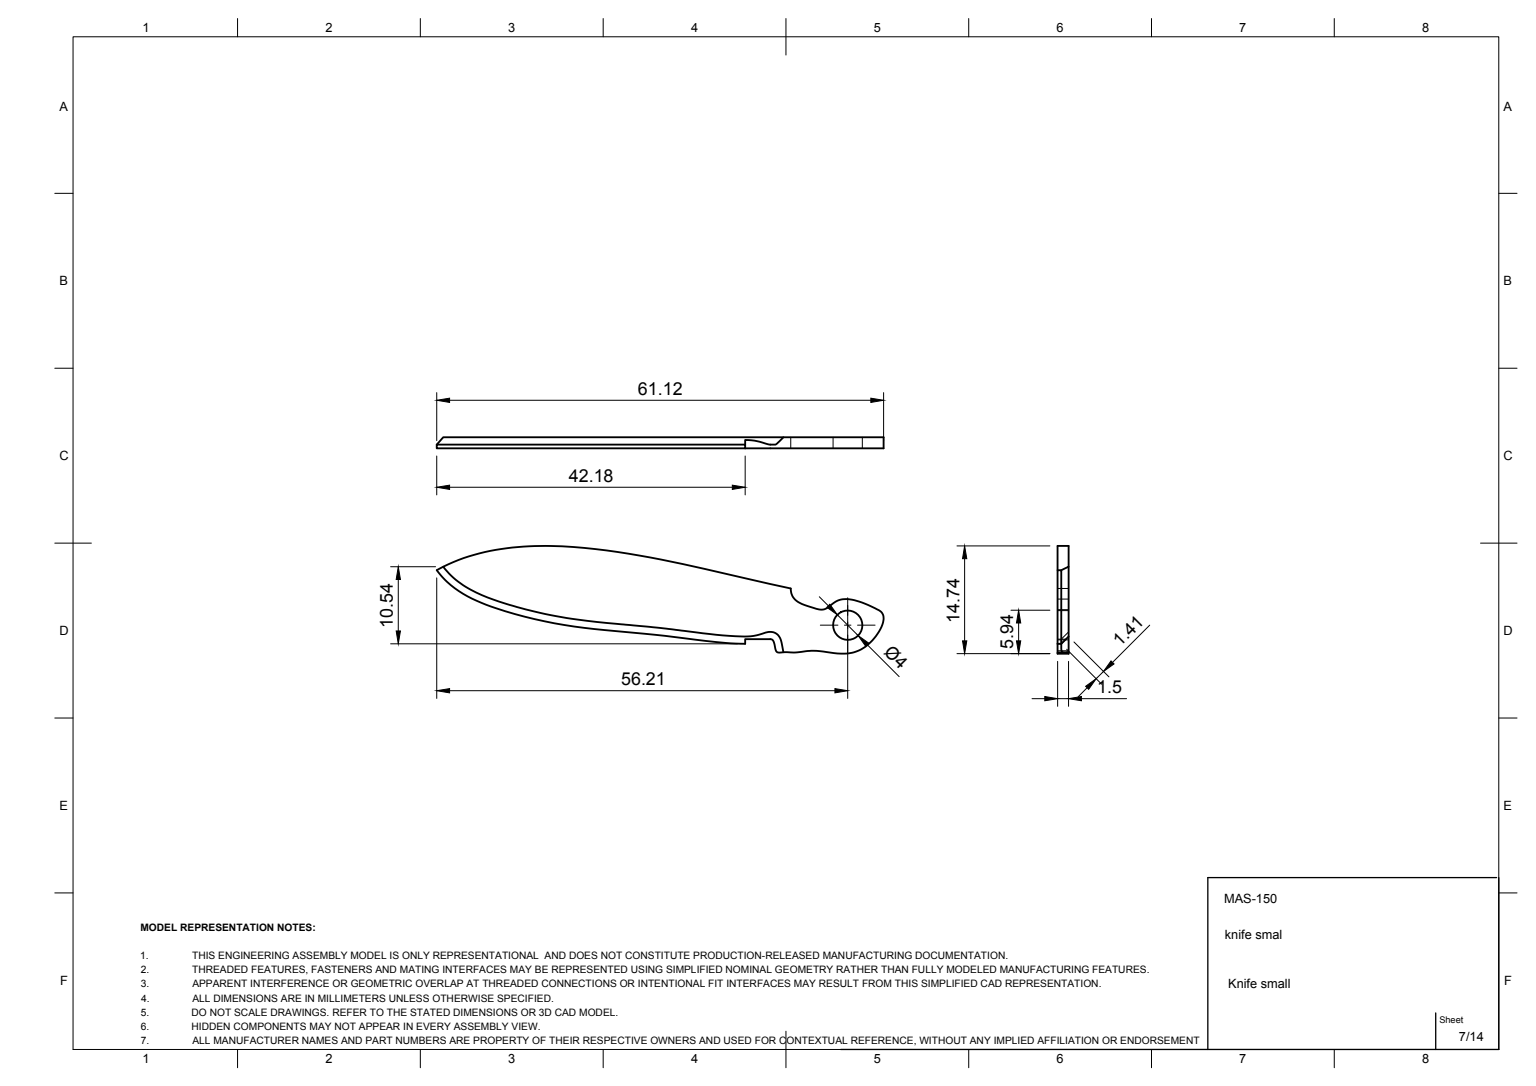
ISO-10303-21;
HEADER;
/* Generated by software containing ST-Developer
 * from STEP Tools, Inc. (www.steptools.com) 
 */

FILE_DESCRIPTION(
/* description */ ('STEP AP203'),
/* implementation_level */ '2;1');

FILE_NAME(
/* name */ 'Knife small.step',
/* time_stamp */ '2026-11-08T21:40:52-08:00',
/* author */ (''),
/* organization */ (''),
/* preprocessor_version */ 'ST-DEVELOPER v20.2',
/* originating_system */ 'Autodesk Translation Framework v15.17.0.0',
/* authorisation */ '');

FILE_SCHEMA (('AUTOMOTIVE_DESIGN { 1 0 10303 214 3 1 1 }'));
ENDSEC;

DATA;
#10=MECHANICAL_DESIGN_GEOMETRIC_PRESENTATION_REPRESENTATION('',(#185),#12137);
#91=B_SPLINE_CURVE_WITH_KNOTS('',3,(#3645,#3646,#3647,#3648,#3649,#3650,
#3651,#3652),.UNSPECIFIED.,.F.,.F.,(4,1,1,1,1,4),(0.,0.0142399187551309,
0.253552302413509,0.548288200579205,0.757181970713106,0.999999999751732),
 .UNSPECIFIED.);
#92=B_SPLINE_CURVE_WITH_KNOTS('',3,(#3655,#3656,#3657,#3658,#3659,#3660,
#3661,#3662),.UNSPECIFIED.,.F.,.F.,(4,1,1,1,1,4),(0.,0.156258367612318,
0.290685780689375,0.48035435867502,0.63435677163295,0.643520450566124),
 .UNSPECIFIED.);
#93=B_SPLINE_CURVE_WITH_KNOTS('',3,(#3689,#3690,#3691,#3692,#3693,#3694,
#3695,#3696),.UNSPECIFIED.,.F.,.F.,(4,1,1,1,1,4),(0.736469307506587,0.759577826910316,
0.780092040409136,0.810242072545427,0.901462701662728,0.958125874426747),
 .UNSPECIFIED.);
#94=B_SPLINE_CURVE_WITH_KNOTS('',3,(#3698,#3699,#3700,#3701,#3702,#3703,
#3704,#3705,#3706,#3707,#3708,#3709,#3710,#3711,#3712,#3713,#3714,#3715,
#3716,#3717,#3718,#3719,#3720,#3721,#3722,#3723,#3724,#3725,#3726,#3727,
#3728,#3729,#3730,#3731,#3732,#3733,#3734,#3735,#3736,#3737,#3738,#3739,
#3740,#3741,#3742,#3743,#3744,#3745,#3746,#3747,#3748,#3749,#3750,#3751,
#3752,#3753,#3754,#3755,#3756,#3757,#3758,#3759,#3760,#3761,#3762,#3763,
#3764,#3765,#3766,#3767,#3768,#3769,#3770,#3771,#3772,#3773,#3774,#3775,
#3776,#3777,#3778,#3779,#3780,#3781,#3782,#3783,#3784,#3785,#3786,#3787,
#3788,#3789,#3790,#3791,#3792,#3793,#3794,#3795,#3796,#3797,#3798,#3799,
#3800,#3801,#3802,#3803,#3804,#3805,#3806,#3807,#3808,#3809,#3810,#3811,
#3812,#3813,#3814,#3815,#3816,#3817,#3818,#3819,#3820,#3821,#3822,#3823,
#3824,#3825,#3826,#3827,#3828,#3829,#3830),.UNSPECIFIED.,.F.,.F.,(4,3,3,
3,3,3,3,3,3,3,3,3,3,3,3,3,3,3,3,3,3,3,3,3,3,3,3,3,3,3,3,3,3,3,3,3,3,3,3,
3,3,3,3,3,4),(-0.304790736556663,-0.304217640980641,-0.296038101920973,
-0.286515952540819,-0.273360133864138,-0.263801143460453,-0.260204315187458,
-0.252535972236165,-0.245519918591342,-0.239298827086652,-0.23653215327504,
-0.233416187936625,-0.215837477852405,-0.203856027214574,-0.191047566863345,
-0.175753773870387,-0.174731606854691,-0.162449438164595,-0.154804922668266,
-0.148252398403841,-0.141338529588791,-0.14102776216038,-0.126737062057896,
-0.12479373531637,-0.116512797864951,-0.111129032227751,-0.108231860413532,
-0.0915022809864805,-0.0886339189716657,-0.0739698737112559,-0.0661726083847358,
-0.0615130055232586,-0.0515620766849569,-0.0423955634704539,-0.0412018838190183,
-0.035176421754689,-0.0328794524142148,-0.0289001906178499,-0.025349772457395,
-0.0253217992573334,-0.0232012051308284,-0.017145962928431,-0.0130970487849195,
-0.00238990525332499,-9.99999152508124E-7),.UNSPECIFIED.);
#95=B_SPLINE_CURVE_WITH_KNOTS('',3,(#3834,#3835,#3836,#3837,#3838,#3839,
#3840,#3841,#3842,#3843,#3844,#3845),.UNSPECIFIED.,.F.,.F.,(4,1,1,1,1,1,
1,1,1,4),(0.69268150065498,0.69714998216664,0.713058394872634,0.723664003343296,
0.736358399716042,0.759577826910316,0.780092040409136,0.810242072545427,
0.901462701662728,0.958125874426747),.UNSPECIFIED.);
#96=B_SPLINE_CURVE_WITH_KNOTS('',3,(#3860,#3861,#3862,#3863,#3864,#3865),
 .UNSPECIFIED.,.F.,.F.,(4,1,1,4),(0.,0.587279823509184,0.66516934088919,
1.),.UNSPECIFIED.);
#97=B_SPLINE_CURVE_WITH_KNOTS('',3,(#3868,#3869,#3870,#3871,#3872,#3873),
 .UNSPECIFIED.,.F.,.F.,(4,1,1,4),(0.,0.587279823509184,0.66516934088919,
1.),.UNSPECIFIED.);
#98=B_SPLINE_CURVE_WITH_KNOTS('',3,(#3889,#3890,#3891,#3892,#3893,#3894,
#3895),.UNSPECIFIED.,.F.,.F.,(4,3,4),(-0.142199063954041,-0.0695096318207944,
0.),.UNSPECIFIED.);
#99=B_SPLINE_CURVE_WITH_KNOTS('',3,(#3896,#3897,#3898,#3899,#3900,#3901,
#3902),.UNSPECIFIED.,.F.,.F.,(4,1,1,1,4),(0.,0.0866729836098282,0.459841695939614,
0.649673299675604,0.828039681548554),.UNSPECIFIED.);
#100=B_SPLINE_CURVE_WITH_KNOTS('',3,(#3903,#3904,#3905,#3906,#3907,#3908,
#3909),.UNSPECIFIED.,.F.,.F.,(4,1,1,1,4),(0.,0.0866729836098282,0.459841695939614,
0.649673299675604,0.845208563176808),.UNSPECIFIED.);
#101=B_SPLINE_CURVE_WITH_KNOTS('',3,(#3911,#3912,#3913,#3914,#3915,#3916,
#3917,#3918,#3919,#3920,#3921,#3922,#3923,#3924,#3925,#3926,#3927,#3928,
#3929,#3930,#3931,#3932,#3933,#3934,#3935,#3936,#3937,#3938,#3939,#3940,
#3941,#3942,#3943,#3944,#3945,#3946,#3947,#3948,#3949,#3950,#3951,#3952,
#3953,#3954,#3955,#3956,#3957,#3958,#3959,#3960,#3961,#3962,#3963,#3964,
#3965,#3966,#3967,#3968,#3969,#3970,#3971,#3972,#3973,#3974,#3975,#3976,
#3977,#3978,#3979,#3980,#3981,#3982,#3983,#3984,#3985,#3986,#3987,#3988,
#3989,#3990,#3991,#3992,#3993,#3994,#3995,#3996,#3997,#3998,#3999,#4000,
#4001,#4002,#4003,#4004,#4005,#4006,#4007,#4008,#4009,#4010,#4011,#4012,
#4013,#4014,#4015,#4016,#4017,#4018,#4019,#4020,#4021,#4022,#4023,#4024,
#4025,#4026,#4027,#4028,#4029,#4030,#4031,#4032,#4033,#4034,#4035,#4036,
#4037,#4038,#4039,#4040,#4041,#4042,#4043,#4044,#4045,#4046,#4047,#4048,
#4049,#4050,#4051,#4052,#4053,#4054,#4055,#4056,#4057,#4058,#4059,#4060,
#4061,#4062,#4063,#4064,#4065,#4066,#4067,#4068,#4069,#4070,#4071,#4072,
#4073,#4074,#4075,#4076,#4077,#4078,#4079,#4080,#4081,#4082,#4083,#4084,
#4085,#4086,#4087,#4088,#4089,#4090,#4091,#4092,#4093,#4094,#4095,#4096,
#4097,#4098,#4099,#4100,#4101,#4102,#4103,#4104,#4105,#4106,#4107,#4108,
#4109,#4110,#4111,#4112,#4113,#4114,#4115,#4116,#4117,#4118,#4119,#4120,
#4121,#4122,#4123,#4124,#4125,#4126,#4127,#4128,#4129,#4130,#4131,#4132,
#4133,#4134,#4135,#4136,#4137,#4138,#4139,#4140,#4141,#4142,#4143,#4144,
#4145,#4146,#4147,#4148,#4149,#4150,#4151,#4152,#4153,#4154,#4155,#4156,
#4157,#4158,#4159,#4160,#4161,#4162,#4163,#4164,#4165,#4166,#4167,#4168,
#4169,#4170,#4171,#4172,#4173,#4174,#4175,#4176,#4177,#4178,#4179,#4180,
#4181,#4182,#4183,#4184,#4185,#4186,#4187,#4188,#4189,#4190,#4191,#4192,
#4193,#4194,#4195,#4196,#4197,#4198,#4199,#4200,#4201,#4202,#4203,#4204,
#4205,#4206,#4207,#4208,#4209,#4210,#4211,#4212,#4213,#4214,#4215,#4216,
#4217,#4218,#4219,#4220,#4221,#4222,#4223,#4224,#4225,#4226,#4227,#4228,
#4229,#4230,#4231,#4232,#4233,#4234,#4235,#4236,#4237,#4238,#4239,#4240,
#4241,#4242,#4243,#4244,#4245,#4246,#4247,#4248,#4249,#4250,#4251,#4252,
#4253,#4254,#4255,#4256,#4257,#4258,#4259,#4260,#4261,#4262,#4263,#4264,
#4265,#4266,#4267,#4268,#4269,#4270,#4271,#4272,#4273,#4274,#4275,#4276,
#4277,#4278,#4279,#4280,#4281,#4282,#4283,#4284,#4285,#4286,#4287,#4288,
#4289,#4290,#4291,#4292,#4293,#4294,#4295),.UNSPECIFIED.,.F.,.F.,(4,3,3,
3,3,3,3,3,3,3,3,3,3,3,3,3,3,3,3,3,3,3,3,3,3,3,3,3,3,3,3,3,3,3,3,3,3,3,3,
3,3,3,3,3,3,3,3,3,3,3,3,3,3,3,3,3,3,3,3,3,3,3,3,3,3,3,3,3,3,3,3,3,3,3,3,
3,3,3,3,3,3,3,3,3,3,3,3,3,3,3,3,3,3,3,3,3,3,3,3,3,3,3,3,3,3,3,3,3,3,3,3,
3,3,3,3,3,3,3,3,3,3,3,3,3,3,3,3,3,4),(1.0000001042787E-6,0.0014871514523892,
0.0749567234267537,0.150089270788223,0.172088117470375,0.241130573114261,
0.312711766240772,0.343094857711695,0.381951662220986,0.421803865009944,
0.428901758240627,0.487519881652639,0.514134072896966,0.582840219819151,
0.657390551246057,0.737159327871297,0.831988683331776,0.852127431697674,
0.930562309987346,1.01139670060428,1.02773758699043,1.09799569327158,1.17527352760952,
1.23343415291206,1.25440919300555,1.25852070377139,1.30827982182686,1.36078487138267,
1.41569393131549,1.44625277535225,1.45683103644174,1.46757702369143,1.71074240249359,
1.9046354359037,2.15693173732147,2.4137324042945,2.66821353221044,2.88528820091008,
3.06961454817592,3.31666055499289,3.48038126011738,3.76387952993356,3.9660510033563,
3.99419905100257,4.00387960603785,4.17190313859031,4.47424018327161,4.5876165750271,
4.60600176545457,4.61648429138331,4.81078750052133,5.05617977077072,5.3812513173155,
5.6262534145718,5.84324989753007,6.03270067111654,6.21030165738215,6.38464570243243,
6.53909882881487,6.55898974748272,6.65552179344928,6.67007122930517,6.80699364566742,
6.9441380090924,7.08360518962895,7.23195205145568,7.33124611521517,7.49685632337973,
7.71469057821715,7.90521396436979,7.97306427912083,8.1326038530189,8.26595178400231,
8.39354231526298,8.5151857419584,8.6112225747131,8.67478294951946,8.69472463683432,
8.77994976234092,8.84186629348611,8.89672828572145,8.9515902779568,9.00448857161819,
9.05627744790037,9.10651371084493,9.11661034222362,9.14263302563896,9.15595525428157,
9.17603250358564,9.19697882034037,9.22071837731693,9.24114544445277,9.2872949501813,
9.31590918197957,9.3419598214356,9.36552499840417,9.37905935500493,9.42076096929037,
9.45178040154512,9.46246258357582,9.47817570718829,9.4936471631625,9.50905917788915,
9.52459264913576,9.54063041470408,9.54655850428292,9.56417707996487,9.58322181605694,
9.60106013585175,9.62444511738643,9.64813998687783,9.66423486245875,9.6919586017109,
9.72029263474653,9.72833972832233,9.75167849681345,9.77575531649194,9.79214986652168,
9.82904279829337,9.86641260150116,9.90467666556498,9.93420348302458,9.97272818736647,
10.0146788654693,10.0614145694852,10.0971799068754,10.2459044783698,10.2612321226266,
10.6513279635848),.UNSPECIFIED.);
#102=B_SPLINE_CURVE_WITH_KNOTS('',3,(#4305,#4306,#4307,#4308,#4309,#4310,
#4311,#4312,#4313,#4314,#4315,#4316,#4317,#4318,#4319,#4320,#4321,#4322,
#4323,#4324),.UNSPECIFIED.,.F.,.F.,(4,2,2,2,2,2,2,2,2,4),(9.9999998042934E-7,
0.000855968525488541,0.00182994379593221,0.00396192280934848,0.0107018008494555,
0.093963121684891,0.228860984301384,0.24733539739969,0.253328089464202,
0.258418228284023),.UNSPECIFIED.);
#142=B_SPLINE_SURFACE_WITH_KNOTS('',3,1,((#3625,#3626),(#3627,#3628),(#3629,
#3630),(#3631,#3632),(#3633,#3634),(#3635,#3636),(#3637,#3638),(#3639,#3640)),
 .UNSPECIFIED.,.F.,.F.,.F.,(4,1,1,1,1,4),(2,2),(0.,0.156258367612318,0.290685780689375,
0.48035435867502,0.63435677163295,0.643520450564764),(0.,0.0719999999999998),
 .UNSPECIFIED.);
#143=B_SPLINE_SURFACE_WITH_KNOTS('',3,1,((#3663,#3664),(#3665,#3666),(#3667,
#3668),(#3669,#3670),(#3671,#3672),(#3673,#3674),(#3675,#3676),(#3677,#3678),
(#3679,#3680),(#3681,#3682),(#3683,#3684),(#3685,#3686)),.UNSPECIFIED.,
 .F.,.F.,.F.,(4,1,1,1,1,1,1,1,1,4),(2,2),(0.69108883441235,0.69714998216664,
0.713058394872634,0.723664003343296,0.736358399716042,0.759577826910316,
0.780092040409136,0.810242072545427,0.901462701662728,0.958125874426747),
(0.,0.216),.UNSPECIFIED.);
#144=B_SPLINE_SURFACE_WITH_KNOTS('',3,1,((#3847,#3848),(#3849,#3850),(#3851,
#3852),(#3853,#3854),(#3855,#3856),(#3857,#3858)),.UNSPECIFIED.,.F.,.F.,
 .F.,(4,1,1,4),(2,2),(0.,0.587279823509184,0.66516934088919,1.),(0.,0.216),
 .UNSPECIFIED.);
#145=B_SPLINE_SURFACE_WITH_KNOTS('',3,1,((#3874,#3875),(#3876,#3877),(#3878,
#3879),(#3880,#3881),(#3882,#3883),(#3884,#3885),(#3886,#3887)),
 .UNSPECIFIED.,.F.,.F.,.F.,(4,1,1,1,4),(2,2),(0.,0.0866729836098282,0.459841695939614,
0.649673299675604,0.845208563176808),(0.,0.216),.UNSPECIFIED.);
#146=B_SPLINE_SURFACE_WITH_KNOTS('',1,3,((#4325,#4326,#4327,#4328,#4329,
#4330,#4331,#4332,#4333,#4334,#4335,#4336,#4337,#4338,#4339,#4340,#4341,
#4342,#4343,#4344,#4345,#4346,#4347,#4348,#4349,#4350,#4351,#4352,#4353,
#4354,#4355,#4356,#4357,#4358,#4359,#4360,#4361,#4362,#4363,#4364,#4365,
#4366,#4367,#4368,#4369,#4370,#4371,#4372,#4373,#4374,#4375,#4376,#4377,
#4378,#4379,#4380,#4381,#4382,#4383,#4384,#4385,#4386,#4387,#4388,#4389,
#4390,#4391,#4392,#4393,#4394,#4395,#4396,#4397,#4398,#4399,#4400,#4401,
#4402,#4403,#4404,#4405,#4406,#4407,#4408,#4409,#4410,#4411,#4412,#4413),
(#4414,#4415,#4416,#4417,#4418,#4419,#4420,#4421,#4422,#4423,#4424,#4425,
#4426,#4427,#4428,#4429,#4430,#4431,#4432,#4433,#4434,#4435,#4436,#4437,
#4438,#4439,#4440,#4441,#4442,#4443,#4444,#4445,#4446,#4447,#4448,#4449,
#4450,#4451,#4452,#4453,#4454,#4455,#4456,#4457,#4458,#4459,#4460,#4461,
#4462,#4463,#4464,#4465,#4466,#4467,#4468,#4469,#4470,#4471,#4472,#4473,
#4474,#4475,#4476,#4477,#4478,#4479,#4480,#4481,#4482,#4483,#4484,#4485,
#4486,#4487,#4488,#4489,#4490,#4491,#4492,#4493,#4494,#4495,#4496,#4497,
#4498,#4499,#4500,#4501,#4502),(#4503,#4504,#4505,#4506,#4507,#4508,#4509,
#4510,#4511,#4512,#4513,#4514,#4515,#4516,#4517,#4518,#4519,#4520,#4521,
#4522,#4523,#4524,#4525,#4526,#4527,#4528,#4529,#4530,#4531,#4532,#4533,
#4534,#4535,#4536,#4537,#4538,#4539,#4540,#4541,#4542,#4543,#4544,#4545,
#4546,#4547,#4548,#4549,#4550,#4551,#4552,#4553,#4554,#4555,#4556,#4557,
#4558,#4559,#4560,#4561,#4562,#4563,#4564,#4565,#4566,#4567,#4568,#4569,
#4570,#4571,#4572,#4573,#4574,#4575,#4576,#4577,#4578,#4579,#4580,#4581,
#4582,#4583,#4584,#4585,#4586,#4587,#4588,#4589,#4590,#4591)),
 .UNSPECIFIED.,.F.,.F.,.F.,(2,1,2),(4,2,2,2,2,2,2,2,2,2,2,2,2,2,2,2,2,2,
2,2,2,2,2,2,2,2,2,2,2,2,2,2,2,2,2,2,2,2,2,2,2,2,3,4),(-1.65164793228187E-5,
1.,1.01),(0.00983313761878334,0.0132402569819186,0.0140920368227025,0.0145179267430944,
0.0147308717032903,0.0147841079433393,0.0148373441833883,0.0149438166634863,
0.016647376345054,0.0183509360266216,0.0192027158674054,0.0200544957081893,
0.0234616150713246,0.0251651747528922,0.0268687344344599,0.0302758537975952,
0.0336829731607305,0.0353865328422982,0.0370900925238658,0.0439043312501364,
0.0473114506132717,0.0507185699764071,0.0541256893395424,0.0575328087026777,
0.0579586986230696,0.0583845885434615,0.0592363683842453,0.0600881482250292,
0.0603010931852251,0.0604075656653231,0.0605140381454211,0.060726983105617,
0.060939928065813,0.0613658179862049,0.0617917079065968,0.0622175978269887,
0.0624305427871847,0.0626434877473806,0.0628564327075766,0.0630693776677726,
0.0634952675881645,0.0639211575085564,0.0643470474289483,0.0653812909954315),
 .UNSPECIFIED.);
#163=SHAPE_REPRESENTATION_RELATIONSHIP('SRR','None',#12186,#174);
#174=ADVANCED_BREP_SHAPE_REPRESENTATION('',(#196),#12127);
#185=STYLED_ITEM('',(#12253),#196);
#196=MANIFOLD_SOLID_BREP('Body1',#1830);
#211=FACE_BOUND('',#635,.T.);
#212=FACE_BOUND('',#637,.T.);
#240=PLANE('',#2009);
#241=PLANE('',#2010);
#242=PLANE('',#2011);
#243=PLANE('',#2012);
#297=LINE('',#3623,#391);
#298=LINE('',#3643,#392);
#299=LINE('',#3654,#393);
#300=LINE('',#3832,#394);
#301=LINE('',#3846,#395);
#302=LINE('',#3867,#396);
#303=LINE('',#4298,#397);
#304=LINE('',#4299,#398);
#305=LINE('',#4302,#399);
#306=LINE('',#4303,#400);
#391=VECTOR('',#2275,2.00000000000001);
#392=VECTOR('',#2278,1000.);
#393=VECTOR('',#2279,1000.);
#394=VECTOR('',#2280,1000.);
#395=VECTOR('',#2281,1000.);
#396=VECTOR('',#2282,1000.);
#397=VECTOR('',#2287,1000.);
#398=VECTOR('',#2288,1000.);
#399=VECTOR('',#2291,1000.);
#400=VECTOR('',#2292,10.);
#471=CYLINDRICAL_SURFACE('',#2006,2.00000000000001);
#513=FACE_OUTER_BOUND('',#629,.T.);
#514=FACE_OUTER_BOUND('',#630,.T.);
#515=FACE_OUTER_BOUND('',#631,.T.);
#516=FACE_OUTER_BOUND('',#632,.T.);
#517=FACE_OUTER_BOUND('',#633,.T.);
#518=FACE_OUTER_BOUND('',#634,.T.);
#519=FACE_OUTER_BOUND('',#636,.T.);
#520=FACE_OUTER_BOUND('',#638,.T.);
#521=FACE_OUTER_BOUND('',#639,.T.);
#522=FACE_OUTER_BOUND('',#640,.T.);
#629=EDGE_LOOP('',(#1329,#1330,#1331,#1332));
#630=EDGE_LOOP('',(#1333,#1334,#1335,#1336));
#631=EDGE_LOOP('',(#1337,#1338,#1339,#1340,#1341));
#632=EDGE_LOOP('',(#1342,#1343,#1344,#1345));
#633=EDGE_LOOP('',(#1346,#1347,#1348,#1349,#1350));
#634=EDGE_LOOP('',(#1351,#1352,#1353,#1354));
#635=EDGE_LOOP('',(#1355));
#636=EDGE_LOOP('',(#1356,#1357,#1358,#1359,#1360,#1361));
#637=EDGE_LOOP('',(#1362));
#638=EDGE_LOOP('',(#1363,#1364,#1365,#1366));
#639=EDGE_LOOP('',(#1367,#1368,#1369,#1370));
#640=EDGE_LOOP('',(#1371,#1372,#1373,#1374,#1375,#1376));
#759=CIRCLE('',#2007,2.00000000000001);
#760=CIRCLE('',#2008,2.00000000000001);
#858=VERTEX_POINT('',#3620);
#859=VERTEX_POINT('',#3622);
#860=VERTEX_POINT('',#3641);
#861=VERTEX_POINT('',#3642);
#862=VERTEX_POINT('',#3644);
#863=VERTEX_POINT('',#3653);
#864=VERTEX_POINT('',#3687);
#865=VERTEX_POINT('',#3688);
#866=VERTEX_POINT('',#3697);
#867=VERTEX_POINT('',#3831);
#868=VERTEX_POINT('',#3833);
#869=VERTEX_POINT('',#3859);
#870=VERTEX_POINT('',#3866);
#871=VERTEX_POINT('',#3888);
#872=VERTEX_POINT('',#4297);
#873=VERTEX_POINT('',#4301);
#1034=EDGE_CURVE('',#858,#858,#759,.T.);
#1035=EDGE_CURVE('',#858,#859,#297,.T.);
#1036=EDGE_CURVE('',#859,#859,#760,.T.);
#1037=EDGE_CURVE('',#860,#861,#298,.T.);
#1038=EDGE_CURVE('',#861,#862,#91,.T.);
#1039=EDGE_CURVE('',#862,#863,#299,.T.);
#1040=EDGE_CURVE('',#863,#860,#92,.T.);
#1041=EDGE_CURVE('',#864,#865,#93,.T.);
#1042=EDGE_CURVE('',#864,#866,#94,.T.);
#1043=EDGE_CURVE('',#867,#866,#300,.T.);
#1044=EDGE_CURVE('',#867,#868,#95,.T.);
#1045=EDGE_CURVE('',#865,#868,#301,.T.);
#1046=EDGE_CURVE('',#868,#869,#96,.T.);
#1047=EDGE_CURVE('',#870,#869,#302,.T.);
#1048=EDGE_CURVE('',#865,#870,#97,.T.);
#1049=EDGE_CURVE('',#862,#871,#98,.T.);
#1050=EDGE_CURVE('',#870,#871,#99,.T.);
#1051=EDGE_CURVE('',#869,#863,#100,.T.);
#1052=EDGE_CURVE('',#871,#864,#101,.T.);
#1053=EDGE_CURVE('',#872,#860,#303,.T.);
#1054=EDGE_CURVE('',#867,#872,#304,.T.);
#1055=EDGE_CURVE('',#872,#873,#305,.T.);
#1056=EDGE_CURVE('',#873,#861,#306,.T.);
#1057=EDGE_CURVE('',#866,#873,#102,.T.);
#1329=ORIENTED_EDGE('',*,*,#1034,.F.);
#1330=ORIENTED_EDGE('',*,*,#1035,.T.);
#1331=ORIENTED_EDGE('',*,*,#1036,.T.);
#1332=ORIENTED_EDGE('',*,*,#1035,.F.);
#1333=ORIENTED_EDGE('',*,*,#1037,.T.);
#1334=ORIENTED_EDGE('',*,*,#1038,.T.);
#1335=ORIENTED_EDGE('',*,*,#1039,.T.);
#1336=ORIENTED_EDGE('',*,*,#1040,.T.);
#1337=ORIENTED_EDGE('',*,*,#1041,.F.);
#1338=ORIENTED_EDGE('',*,*,#1042,.T.);
#1339=ORIENTED_EDGE('',*,*,#1043,.F.);
#1340=ORIENTED_EDGE('',*,*,#1044,.T.);
#1341=ORIENTED_EDGE('',*,*,#1045,.F.);
#1342=ORIENTED_EDGE('',*,*,#1046,.T.);
#1343=ORIENTED_EDGE('',*,*,#1047,.F.);
#1344=ORIENTED_EDGE('',*,*,#1048,.F.);
#1345=ORIENTED_EDGE('',*,*,#1045,.T.);
#1346=ORIENTED_EDGE('',*,*,#1039,.F.);
#1347=ORIENTED_EDGE('',*,*,#1049,.T.);
#1348=ORIENTED_EDGE('',*,*,#1050,.F.);
#1349=ORIENTED_EDGE('',*,*,#1047,.T.);
#1350=ORIENTED_EDGE('',*,*,#1051,.T.);
#1351=ORIENTED_EDGE('',*,*,#1050,.T.);
#1352=ORIENTED_EDGE('',*,*,#1052,.T.);
#1353=ORIENTED_EDGE('',*,*,#1041,.T.);
#1354=ORIENTED_EDGE('',*,*,#1048,.T.);
#1355=ORIENTED_EDGE('',*,*,#1036,.F.);
#1356=ORIENTED_EDGE('',*,*,#1053,.T.);
#1357=ORIENTED_EDGE('',*,*,#1040,.F.);
#1358=ORIENTED_EDGE('',*,*,#1051,.F.);
#1359=ORIENTED_EDGE('',*,*,#1046,.F.);
#1360=ORIENTED_EDGE('',*,*,#1044,.F.);
#1361=ORIENTED_EDGE('',*,*,#1054,.T.);
#1362=ORIENTED_EDGE('',*,*,#1034,.T.);
#1363=ORIENTED_EDGE('',*,*,#1055,.T.);
#1364=ORIENTED_EDGE('',*,*,#1056,.T.);
#1365=ORIENTED_EDGE('',*,*,#1037,.F.);
#1366=ORIENTED_EDGE('',*,*,#1053,.F.);
#1367=ORIENTED_EDGE('',*,*,#1043,.T.);
#1368=ORIENTED_EDGE('',*,*,#1057,.T.);
#1369=ORIENTED_EDGE('',*,*,#1055,.F.);
#1370=ORIENTED_EDGE('',*,*,#1054,.F.);
#1371=ORIENTED_EDGE('',*,*,#1042,.F.);
#1372=ORIENTED_EDGE('',*,*,#1052,.F.);
#1373=ORIENTED_EDGE('',*,*,#1049,.F.);
#1374=ORIENTED_EDGE('',*,*,#1038,.F.);
#1375=ORIENTED_EDGE('',*,*,#1056,.F.);
#1376=ORIENTED_EDGE('',*,*,#1057,.F.);
#1741=ADVANCED_FACE('',(#513),#471,.F.);
#1742=ADVANCED_FACE('',(#514),#142,.F.);
#1743=ADVANCED_FACE('',(#515),#143,.F.);
#1744=ADVANCED_FACE('',(#516),#144,.F.);
#1745=ADVANCED_FACE('',(#517),#145,.F.);
#1746=ADVANCED_FACE('',(#518,#211),#240,.F.);
#1747=ADVANCED_FACE('',(#519,#212),#241,.T.);
#1748=ADVANCED_FACE('',(#520),#242,.F.);
#1749=ADVANCED_FACE('',(#521),#243,.F.);
#1750=ADVANCED_FACE('',(#522),#146,.T.);
#1830=CLOSED_SHELL('',(#1741,#1742,#1743,#1744,#1745,#1746,#1747,#1748,
#1749,#1750));
#2005=AXIS2_PLACEMENT_3D('',#3618,#2269,#2270);
#2006=AXIS2_PLACEMENT_3D('',#3619,#2271,#2272);
#2007=AXIS2_PLACEMENT_3D('',#3621,#2273,#2274);
#2008=AXIS2_PLACEMENT_3D('',#3624,#2276,#2277);
#2009=AXIS2_PLACEMENT_3D('',#3910,#2283,#2284);
#2010=AXIS2_PLACEMENT_3D('',#4296,#2285,#2286);
#2011=AXIS2_PLACEMENT_3D('',#4300,#2289,#2290);
#2012=AXIS2_PLACEMENT_3D('',#4304,#2293,#2294);
#2269=DIRECTION('axis',(0.,0.,1.));
#2270=DIRECTION('refdir',(1.,0.,0.));
#2271=DIRECTION('center_axis',(0.,1.,0.));
#2272=DIRECTION('ref_axis',(0.,0.,1.));
#2273=DIRECTION('center_axis',(0.,1.,0.));
#2274=DIRECTION('ref_axis',(0.,0.,1.));
#2275=DIRECTION('',(0.,1.,0.));
#2276=DIRECTION('center_axis',(0.,1.,0.));
#2277=DIRECTION('ref_axis',(0.,0.,1.));
#2278=DIRECTION('',(0.,1.,0.));
#2279=DIRECTION('',(0.,-1.,0.));
#2280=DIRECTION('',(0.,1.,0.));
#2281=DIRECTION('',(0.,-1.,0.));
#2282=DIRECTION('',(0.,-1.,0.));
#2283=DIRECTION('center_axis',(0.,-1.,0.));
#2284=DIRECTION('ref_axis',(5.55111512312576E-17,0.,-1.));
#2285=DIRECTION('center_axis',(0.,-1.,0.));
#2286=DIRECTION('ref_axis',(5.55111512312576E-17,0.,-1.));
#2287=DIRECTION('',(0.211715251599179,0.,0.977331393254251));
#2288=DIRECTION('',(-0.977331393254251,0.,0.211715251599179));
#2289=DIRECTION('center_axis',(-0.977331393254252,0.,0.211715251599179));
#2290=DIRECTION('ref_axis',(0.211715251599179,0.,0.977331393254252));
#2291=DIRECTION('',(0.,1.,0.));
#2292=DIRECTION('',(0.149706258215497,-0.707102223259955,0.691082109529645));
#2293=DIRECTION('center_axis',(-0.211715251599179,0.,-0.977331393254252));
#2294=DIRECTION('ref_axis',(-0.977331393254252,0.,0.211715251599179));
#3618=CARTESIAN_POINT('',(0.,0.,0.));
#3619=CARTESIAN_POINT('Origin',(25.5182217655705,0.,-1.87222413531758));
#3620=CARTESIAN_POINT('',(25.5182217655705,0.,-3.87222413531759));
#3621=CARTESIAN_POINT('Origin',(25.5182217655705,0.,-1.87222413531758));
#3622=CARTESIAN_POINT('',(25.5182217655705,1.5,-3.87222413531759));
#3623=CARTESIAN_POINT('',(25.5182217655705,0.,-3.87222413531759));
#3624=CARTESIAN_POINT('Origin',(25.5182217655705,1.5,-1.87222413531758));
#3625=CARTESIAN_POINT('Ctrl Pts',(-31.0084166862739,0.499999999999999,2.67704093130204));
#3626=CARTESIAN_POINT('Ctrl Pts',(-31.0084166862739,-0.219999999999999,
2.67704093130204));
#3627=CARTESIAN_POINT('Ctrl Pts',(-28.2076463187592,0.499999999999999,5.17696258174617));
#3628=CARTESIAN_POINT('Ctrl Pts',(-28.2076463187592,-0.219999999999999,
5.17696258174617));
#3629=CARTESIAN_POINT('Ctrl Pts',(-21.482456130384,0.499999999999999,6.37819210999435));
#3630=CARTESIAN_POINT('Ctrl Pts',(-21.482456130384,-0.219999999999999,6.37819210999435));
#3631=CARTESIAN_POINT('Ctrl Pts',(-10.4420666215006,0.499999999999999,6.51321702489205));
#3632=CARTESIAN_POINT('Ctrl Pts',(-10.4420666215006,-0.219999999999999,
6.51321702489205));
#3633=CARTESIAN_POINT('Ctrl Pts',(0.282701922195941,0.499999999999999,4.72397216873886));
#3634=CARTESIAN_POINT('Ctrl Pts',(0.282701922195941,-0.219999999999999,
4.72397216873886));
#3635=CARTESIAN_POINT('Ctrl Pts',(8.69351499070982,0.499999999999999,4.31367676768492));
#3636=CARTESIAN_POINT('Ctrl Pts',(8.69351499070982,-0.219999999999999,4.31367676768492));
#3637=CARTESIAN_POINT('Ctrl Pts',(12.1517585870304,0.499999999999999,3.62923948763913));
#3638=CARTESIAN_POINT('Ctrl Pts',(12.1517585870304,-0.219999999999999,3.62923948763913));
#3639=CARTESIAN_POINT('Ctrl Pts',(12.3457959310433,0.499999999999999,3.58626341940775));
#3640=CARTESIAN_POINT('Ctrl Pts',(12.3457959310433,-0.219999999999999,3.58626341940775));
#3641=CARTESIAN_POINT('',(12.3457959311297,0.,3.58626341938894));
#3642=CARTESIAN_POINT('',(12.3457959979746,0.500000312196434,3.58626372434223));
#3643=CARTESIAN_POINT('',(12.3457959311296,1.5,3.58626341938861));
#3644=CARTESIAN_POINT('',(-31.0084166020303,0.499999717221561,2.67704086144519));
#3645=CARTESIAN_POINT('Ctrl Pts',(12.3457959311296,0.499999999999999,3.58626341938861));
#3646=CARTESIAN_POINT('Ctrl Pts',(12.1517585870946,0.499999999999999,3.62923948762642));
#3647=CARTESIAN_POINT('Ctrl Pts',(8.69351499074593,0.499999999999999,4.31367676768316));
#3648=CARTESIAN_POINT('Ctrl Pts',(0.282701922195941,0.499999999999999,4.72397216873886));
#3649=CARTESIAN_POINT('Ctrl Pts',(-10.4420666215006,0.499999999999999,6.51321702489205));
#3650=CARTESIAN_POINT('Ctrl Pts',(-21.4824561267119,0.499999999999999,6.37819211003926));
#3651=CARTESIAN_POINT('Ctrl Pts',(-28.2076463113667,0.499999999999999,5.1769625830666));
#3652=CARTESIAN_POINT('Ctrl Pts',(-31.008416677683,0.499999994355063,2.67704093897015));
#3653=CARTESIAN_POINT('',(-31.0084166862739,0.,2.67704093130204));
#3654=CARTESIAN_POINT('',(-31.0084166862739,1.5,2.67704093130204));
#3655=CARTESIAN_POINT('Ctrl Pts',(-31.0084166862739,0.,2.67704093130204));
#3656=CARTESIAN_POINT('Ctrl Pts',(-28.2076463187592,0.,5.17696258174617));
#3657=CARTESIAN_POINT('Ctrl Pts',(-21.482456130384,0.,6.37819210999435));
#3658=CARTESIAN_POINT('Ctrl Pts',(-10.4420666215006,0.,6.51321702489205));
#3659=CARTESIAN_POINT('Ctrl Pts',(0.282701922195941,0.,4.72397216873886));
#3660=CARTESIAN_POINT('Ctrl Pts',(8.69351499074223,0.,4.31367676768334));
#3661=CARTESIAN_POINT('Ctrl Pts',(12.151758587088,0.,3.62923948762772));
#3662=CARTESIAN_POINT('Ctrl Pts',(12.3457959311297,0.,3.58626341938894));
#3663=CARTESIAN_POINT('Ctrl Pts',(15.4777909450074,1.5,2.26366898793832));
#3664=CARTESIAN_POINT('Ctrl Pts',(15.4777909450074,-0.660000000000002,2.26366898793832));
#3665=CARTESIAN_POINT('Ctrl Pts',(15.604589304325,1.5,2.22082970559645));
#3666=CARTESIAN_POINT('Ctrl Pts',(15.604589304325,-0.660000000000002,2.22082970559645));
#3667=CARTESIAN_POINT('Ctrl Pts',(16.0321425201824,1.5,2.16989877476718));
#3668=CARTESIAN_POINT('Ctrl Pts',(16.0321425201824,-0.660000000000002,2.16989877476718));
#3669=CARTESIAN_POINT('Ctrl Pts',(16.380711317993,1.5,3.03159825743662));
#3670=CARTESIAN_POINT('Ctrl Pts',(16.380711317993,-0.660000000000002,3.03159825743662));
#3671=CARTESIAN_POINT('Ctrl Pts',(16.7818328065524,1.5,3.98512327200762));
#3672=CARTESIAN_POINT('Ctrl Pts',(16.7818328065524,-0.660000000000002,3.98512327200762));
#3673=CARTESIAN_POINT('Ctrl Pts',(18.0021442434375,1.5,3.42330192479396));
#3674=CARTESIAN_POINT('Ctrl Pts',(18.0021442434375,-0.660000000000002,3.42330192479396));
#3675=CARTESIAN_POINT('Ctrl Pts',(19.1270049692968,1.5,3.45147463333956));
#3676=CARTESIAN_POINT('Ctrl Pts',(19.1270049692968,-0.660000000000002,3.45147463333956));
#3677=CARTESIAN_POINT('Ctrl Pts',(21.1106762553254,1.5,2.59215126849901));
#3678=CARTESIAN_POINT('Ctrl Pts',(21.1106762553254,-0.660000000000002,2.59215126849901));
#3679=CARTESIAN_POINT('Ctrl Pts',(24.1154409179203,1.5,2.13122905062585));
#3680=CARTESIAN_POINT('Ctrl Pts',(24.1154409179203,-0.660000000000002,2.13122905062585));
#3681=CARTESIAN_POINT('Ctrl Pts',(28.7570716465227,1.5,2.48541219309353));
#3682=CARTESIAN_POINT('Ctrl Pts',(28.7570716465227,-0.660000000000002,2.48541219309353));
#3683=CARTESIAN_POINT('Ctrl Pts',(30.8610725977064,1.5,-4.32380575261494));
#3684=CARTESIAN_POINT('Ctrl Pts',(30.8610725977064,-0.660000000000002,-4.32380575261494));
#3685=CARTESIAN_POINT('Ctrl Pts',(29.2519383950227,1.5,-4.7724535583603));
#3686=CARTESIAN_POINT('Ctrl Pts',(29.2519383950227,-0.660000000000002,-4.7724535583603));
#3687=CARTESIAN_POINT('',(17.7057705722702,1.5,3.60431887284736));
#3688=CARTESIAN_POINT('',(29.2519383950227,1.5,-4.77245355836028));
#3689=CARTESIAN_POINT('Ctrl Pts',(17.7057705722702,1.5,3.60431887284736));
#3690=CARTESIAN_POINT('Ctrl Pts',(18.2596235045177,1.5,3.42974716334014));
#3691=CARTESIAN_POINT('Ctrl Pts',(19.1299826853614,1.5,3.45018469129812));
#3692=CARTESIAN_POINT('Ctrl Pts',(21.1106762553254,1.5,2.59215126849901));
#3693=CARTESIAN_POINT('Ctrl Pts',(24.1154409179203,1.5,2.13122905062585));
#3694=CARTESIAN_POINT('Ctrl Pts',(28.7570716465227,1.5,2.48541219309353));
#3695=CARTESIAN_POINT('Ctrl Pts',(30.8610725977064,1.5,-4.32380575261494));
#3696=CARTESIAN_POINT('Ctrl Pts',(29.2519383950227,1.5,-4.77245355836028));
#3697=CARTESIAN_POINT('',(15.5758189333363,0.50000155332938,2.23621039387092));
#3698=CARTESIAN_POINT('Ctrl Pts',(17.7057705722709,1.49999999999931,3.60431887284718));
#3699=CARTESIAN_POINT('Ctrl Pts',(17.7031110290994,1.49722275297065,3.6051571477229));
#3700=CARTESIAN_POINT('Ctrl Pts',(17.7004506633562,1.49444326036002,3.6059992825549));
#3701=CARTESIAN_POINT('Ctrl Pts',(17.6977896002535,1.491661645525,3.60684525708301));
#3702=CARTESIAN_POINT('Ctrl Pts',(17.6598094264402,1.45196089028633,3.61891947643783));
#3703=CARTESIAN_POINT('Ctrl Pts',(17.6216545449597,1.41182941608976,3.63178245853097));
#3704=CARTESIAN_POINT('Ctrl Pts',(17.5835382242194,1.37164748726708,3.64484827643156));
#3705=CARTESIAN_POINT('Ctrl Pts',(17.5391653937624,1.32486999456962,3.66005875087463));
#3706=CARTESIAN_POINT('Ctrl Pts',(17.4948445411659,1.27802412435748,3.67554478384865));
#3707=CARTESIAN_POINT('Ctrl Pts',(17.4508805310589,1.23170981145215,3.69044990780328));
#3708=CARTESIAN_POINT('Ctrl Pts',(17.390139775776,1.16772187360406,3.71104285381494));
#3709=CARTESIAN_POINT('Ctrl Pts',(17.3300783592064,1.10474858484553,3.73053128190524));
#3710=CARTESIAN_POINT('Ctrl Pts',(17.2714557074252,1.04437211368676,3.746748229346));
#3711=CARTESIAN_POINT('Ctrl Pts',(17.2288606109445,1.00050269570534,3.75853142952328));
#3712=CARTESIAN_POINT('Ctrl Pts',(17.1870235802448,0.958004253366488,3.76859067496704));
#3713=CARTESIAN_POINT('Ctrl Pts',(17.1462434201237,0.91748371187863,3.77607540849513));
#3714=CARTESIAN_POINT('Ctrl Pts',(17.1308987836395,0.902236763915967,3.77889174160487));
#3715=CARTESIAN_POINT('Ctrl Pts',(17.115703959382,0.8872698558268,3.78134315103857));
#3716=CARTESIAN_POINT('Ctrl Pts',(17.1006757019891,0.872615321519951,3.78338238638474));
#3717=CARTESIAN_POINT('Ctrl Pts',(17.0686358538502,0.841372241137127,3.7877299823237));
#3718=CARTESIAN_POINT('Ctrl Pts',(17.0368320316669,0.81103299831122,3.79027827290231));
#3719=CARTESIAN_POINT('Ctrl Pts',(17.0056623734324,0.782246495163689,3.79033388695513));
#3720=CARTESIAN_POINT('Ctrl Pts',(16.9771440878453,0.755908647259284,3.79038477033117));
#3721=CARTESIAN_POINT('Ctrl Pts',(16.9491574377736,0.730870613915962,3.78834731258798));
#3722=CARTESIAN_POINT('Ctrl Pts',(16.9220198105467,0.707629391615289,3.78366412357332));
#3723=CARTESIAN_POINT('Ctrl Pts',(16.8979570438198,0.687021543110594,3.77951156875136));
#3724=CARTESIAN_POINT('Ctrl Pts',(16.8773111036014,0.670182282643359,3.77375218638167));
#3725=CARTESIAN_POINT('Ctrl Pts',(16.8596132434589,0.656301257240817,3.7673887064672));
#3726=CARTESIAN_POINT('Ctrl Pts',(16.8517425657586,0.650128020690516,3.7645587089954));
#3727=CARTESIAN_POINT('Ctrl Pts',(16.8444549751791,0.644539864366037,3.76160908956875));
#3728=CARTESIAN_POINT('Ctrl Pts',(16.8377108992226,0.639465511443471,3.75862385138259));
#3729=CARTESIAN_POINT('Ctrl Pts',(16.8301153862163,0.633750523375398,3.75526172799965));
#3730=CARTESIAN_POINT('Ctrl Pts',(16.823208377781,0.628687637778199,3.75185624556522));
#3731=CARTESIAN_POINT('Ctrl Pts',(16.8169313605122,0.624174347799258,3.74853336303511));
#3732=CARTESIAN_POINT('Ctrl Pts',(16.7815195844566,0.598712634510066,3.72978733016992));
#3733=CARTESIAN_POINT('Ctrl Pts',(16.7484971453216,0.578077766495358,3.70423315774478));
#3734=CARTESIAN_POINT('Ctrl Pts',(16.7173105344503,0.561525876955449,3.67247601143094));
#3735=CARTESIAN_POINT('Ctrl Pts',(16.6960540920307,0.550244295625811,3.65083069848507));
#3736=CARTESIAN_POINT('Ctrl Pts',(16.6761897156968,0.541152670171255,3.62684519200596));
#3737=CARTESIAN_POINT('Ctrl Pts',(16.6575806498602,0.533786696249175,3.6013739187025));
#3738=CARTESIAN_POINT('Ctrl Pts',(16.6376871086567,0.525912292073837,3.57414451184149));
#3739=CARTESIAN_POINT('Ctrl Pts',(16.619225449201,0.520009984352785,3.54522278492793));
#3740=CARTESIAN_POINT('Ctrl Pts',(16.602024489444,0.515512535079858,3.51567962967423));
#3741=CARTESIAN_POINT('Ctrl Pts',(16.5814858836639,0.51014240812546,3.48040396902344));
#3742=CARTESIAN_POINT('Ctrl Pts',(16.5622765757694,0.506656585391937,3.44342095261399));
#3743=CARTESIAN_POINT('Ctrl Pts',(16.5443411772826,0.504350243957675,3.40642785852021));
#3744=CARTESIAN_POINT('Ctrl Pts',(16.5431424574651,0.50419609866866,3.40395540969025));
#3745=CARTESIAN_POINT('Ctrl Pts',(16.5419494305495,0.504047222090552,3.40148292861609));
#3746=CARTESIAN_POINT('Ctrl Pts',(16.5407620833152,0.503903403797068,3.39901092252946));
#3747=CARTESIAN_POINT('Ctrl Pts',(16.5264951398497,0.502175309939439,3.36930775730037));
#3748=CARTESIAN_POINT('Ctrl Pts',(16.5126214116979,0.501131296660439,3.33877520325719));
#3749=CARTESIAN_POINT('Ctrl Pts',(16.4992129271919,0.500508072838966,3.30825796373013));
#3750=CARTESIAN_POINT('Ctrl Pts',(16.4908673841387,0.500120173577757,3.28926380102513));
#3751=CARTESIAN_POINT('Ctrl Pts',(16.4827014884031,0.499895284473406,3.27027731286861));
#3752=CARTESIAN_POINT('Ctrl Pts',(16.4747329295069,0.499769922015154,3.25150626308357));
#3753=CARTESIAN_POINT('Ctrl Pts',(16.4679026502636,0.499662467128061,3.23541658948106));
#3754=CARTESIAN_POINT('Ctrl Pts',(16.4608038217544,0.499628622524833,3.21850215242504));
#3755=CARTESIAN_POINT('Ctrl Pts',(16.4538691941752,0.499633152943755,3.20186981087292));
#3756=CARTESIAN_POINT('Ctrl Pts',(16.4465521506316,0.499637933196501,3.18432026463122));
#3757=CARTESIAN_POINT('Ctrl Pts',(16.4394159727634,0.499685437619131,3.16708885086712));
#3758=CARTESIAN_POINT('Ctrl Pts',(16.4329679810904,0.499734274346846,3.1515094741843));
#3759=CARTESIAN_POINT('Ctrl Pts',(16.4326781541,0.499736469480235,3.15080920593255));
#3760=CARTESIAN_POINT('Ctrl Pts',(16.4323897151146,0.499738665310908,3.15011226221279));
#3761=CARTESIAN_POINT('Ctrl Pts',(16.4321027118697,0.499740859977208,3.14941876225688));
#3762=CARTESIAN_POINT('Ctrl Pts',(16.4189048123257,0.499841782130048,3.11752803309743));
#3763=CARTESIAN_POINT('Ctrl Pts',(16.4056285637068,0.499964068050572,3.08539406439388));
#3764=CARTESIAN_POINT('Ctrl Pts',(16.3923146363802,0.499993418608882,3.05341112999197));
#3765=CARTESIAN_POINT('Ctrl Pts',(16.3905041364871,0.499997409856647,3.04906191747964));
#3766=CARTESIAN_POINT('Ctrl Pts',(16.3885584669575,0.500000000000007,3.04439241037328));
#3767=CARTESIAN_POINT('Ctrl Pts',(16.386497303637,0.500000000000006,3.03945284932727));
#3768=CARTESIAN_POINT('Ctrl Pts',(16.3777142389215,0.500000000000002,3.01840430654475));
#3769=CARTESIAN_POINT('Ctrl Pts',(16.3668279599517,0.500013565738278,2.99243842907649));
#3770=CARTESIAN_POINT('Ctrl Pts',(16.355357683933,0.500028207045904,2.96547257823315));
#3771=CARTESIAN_POINT('Ctrl Pts',(16.3479004028895,0.500037725940273,2.94794100985699));
#3772=CARTESIAN_POINT('Ctrl Pts',(16.3401961527186,0.500047699457953,2.9299898633552));
#3773=CARTESIAN_POINT('Ctrl Pts',(16.3326784228899,0.500054695275253,2.91267644838095));
#3774=CARTESIAN_POINT('Ctrl Pts',(16.3286328985424,0.500058459942229,2.90335956104754));
#3775=CARTESIAN_POINT('Ctrl Pts',(16.3246417171666,0.500061362311546,2.89422674409416));
#3776=CARTESIAN_POINT('Ctrl Pts',(16.3207751647991,0.500062867507892,2.88543672368119));
#3777=CARTESIAN_POINT('Ctrl Pts',(16.2984479439476,0.500071559191861,2.83467917318227));
#3778=CARTESIAN_POINT('Ctrl Pts',(16.2750727227244,0.500028068253373,2.78349236485305));
#3779=CARTESIAN_POINT('Ctrl Pts',(16.2507208369999,0.500006270829282,2.73363070383891));
#3780=CARTESIAN_POINT('Ctrl Pts',(16.2465455961156,0.500002533562391,2.72508169667038));
#3781=CARTESIAN_POINT('Ctrl Pts',(16.2423066128638,0.500000000000009,2.71649975941386));
#3782=CARTESIAN_POINT('Ctrl Pts',(16.2380046463533,0.500000000000007,2.7078994039198));
#3783=CARTESIAN_POINT('Ctrl Pts',(16.2160115257873,0.499999999999997,2.66393145232615));
#3784=CARTESIAN_POINT('Ctrl Pts',(16.1923725125796,0.500031011240663,2.61947930368824));
#3785=CARTESIAN_POINT('Ctrl Pts',(16.1671669155192,0.500038395999784,2.57649896923451));
#3786=CARTESIAN_POINT('Ctrl Pts',(16.1537644249716,0.50004232267385,2.55364517510015));
#3787=CARTESIAN_POINT('Ctrl Pts',(16.1399190089963,0.500039569353616,2.53120874899483));
#3788=CARTESIAN_POINT('Ctrl Pts',(16.125647161097,0.500021921973862,2.50947625132159));
#3789=CARTESIAN_POINT('Ctrl Pts',(16.1171183833107,0.500011375996811,2.49648903027618));
#3790=CARTESIAN_POINT('Ctrl Pts',(16.108310702811,0.499999999999986,2.48355951018343));
#3791=CARTESIAN_POINT('Ctrl Pts',(16.0992240534471,0.49999999999999,2.47078446108149));
#3792=CARTESIAN_POINT('Ctrl Pts',(16.0798188371901,0.499999999999998,2.44350239256654));
#3793=CARTESIAN_POINT('Ctrl Pts',(16.0591401886511,0.500032153485344,2.41692570967048));
#3794=CARTESIAN_POINT('Ctrl Pts',(16.0371885635348,0.500034626496161,2.39199625974152));
#3795=CARTESIAN_POINT('Ctrl Pts',(16.0169673495177,0.500036904563537,2.36903195802482));
#3796=CARTESIAN_POINT('Ctrl Pts',(15.9952885015027,0.50000000000003,2.34703350101923));
#3797=CARTESIAN_POINT('Ctrl Pts',(15.9721147607565,0.500000000000017,2.32697564309227));
#3798=CARTESIAN_POINT('Ctrl Pts',(15.9690970350271,0.500000000000016,2.3243636731645));
#3799=CARTESIAN_POINT('Ctrl Pts',(15.9660539660289,0.499999447831871,2.32178460547913));
#3800=CARTESIAN_POINT('Ctrl Pts',(15.9629854828687,0.499998755868987,2.31924057762361));
#3801=CARTESIAN_POINT('Ctrl Pts',(15.9474963783552,0.49999526297531,2.30639882119796));
#3802=CARTESIAN_POINT('Ctrl Pts',(15.9312993972364,0.500000000000034,2.2943997687265));
#3803=CARTESIAN_POINT('Ctrl Pts',(15.9143698160608,0.500000000000026,2.28353887216815));
#3804=CARTESIAN_POINT('Ctrl Pts',(15.9079160821409,0.500000000000023,2.2793985844793));
#3805=CARTESIAN_POINT('Ctrl Pts',(15.9013558869196,0.500000796710013,2.27542369857025));
#3806=CARTESIAN_POINT('Ctrl Pts',(15.8946878996606,0.50000115650804,2.27163051661969));
#3807=CARTESIAN_POINT('Ctrl Pts',(15.8831363014348,0.500001779820908,2.26505922123644));
#3808=CARTESIAN_POINT('Ctrl Pts',(15.8713127070406,0.500000000000019,2.25906251116108));
#3809=CARTESIAN_POINT('Ctrl Pts',(15.8592065464433,0.500000000000015,2.25370333364518));
#3810=CARTESIAN_POINT('Ctrl Pts',(15.8484050624903,0.500000000000012,2.24892171279406));
#3811=CARTESIAN_POINT('Ctrl Pts',(15.8373786323162,0.499983033802094,2.24464763132202));
#3812=CARTESIAN_POINT('Ctrl Pts',(15.8261197469387,0.499988596289819,2.24092577040655));
#3813=CARTESIAN_POINT('Ctrl Pts',(15.8260310399079,0.499988640115806,2.24089644643532));
#3814=CARTESIAN_POINT('Ctrl Pts',(15.8259423255587,0.499988684421491,2.24086715909388));
#3815=CARTESIAN_POINT('Ctrl Pts',(15.8258536038921,0.499988729180149,2.24083790838682));
#3816=CARTESIAN_POINT('Ctrl Pts',(15.8191277861575,0.49999212224741,2.23862046892895));
#3817=CARTESIAN_POINT('Ctrl Pts',(15.8123599112164,0.499999999999994,2.23661356904048));
#3818=CARTESIAN_POINT('Ctrl Pts',(15.8055540048929,0.499999999999989,2.23480861085287));
#3819=CARTESIAN_POINT('Ctrl Pts',(15.7861201063075,0.499999999999977,2.22965465005735));
#3820=CARTESIAN_POINT('Ctrl Pts',(15.7663760877143,0.499999999999995,2.22614752151095));
#3821=CARTESIAN_POINT('Ctrl Pts',(15.7464171834751,0.499999999999999,2.22408394272492));
#3822=CARTESIAN_POINT('Ctrl Pts',(15.7330714101828,0.500000000000001,2.22270410471783));
#3823=CARTESIAN_POINT('Ctrl Pts',(15.7196296183475,0.499965185715635,2.22196957770925));
#3824=CARTESIAN_POINT('Ctrl Pts',(15.7061201902805,0.499946779332921,2.22181911498421));
#3825=CARTESIAN_POINT('Ctrl Pts',(15.6703952081703,0.499898104608135,2.22142122410876));
#3826=CARTESIAN_POINT('Ctrl Pts',(15.6345058507886,0.500000000000026,2.22511547817362));
#3827=CARTESIAN_POINT('Ctrl Pts',(15.5992847698687,0.500000000000013,2.23152789104314));
#3828=CARTESIAN_POINT('Ctrl Pts',(15.5914264811459,0.50000000000001,2.23295858511675));
#3829=CARTESIAN_POINT('Ctrl Pts',(15.5836014534938,0.500000633198017,2.23452449876141));
#3830=CARTESIAN_POINT('Ctrl Pts',(15.5758189333363,0.50000155333021,2.23621039387093));
#3831=CARTESIAN_POINT('',(15.5758189333363,0.,2.23621039387092));
#3832=CARTESIAN_POINT('',(15.5758189333363,0.,2.23621039387092));
#3833=CARTESIAN_POINT('',(29.2519383950227,0.,-4.77245355836028));
#3834=CARTESIAN_POINT('Ctrl Pts',(15.5758189333363,0.,2.23621039387092));
#3835=CARTESIAN_POINT('Ctrl Pts',(15.6655680769744,0.,2.21676717105701));
#3836=CARTESIAN_POINT('Ctrl Pts',(16.0491847574363,0.,2.21202901452892));
#3837=CARTESIAN_POINT('Ctrl Pts',(16.380711317993,0.,3.03159825743662));
#3838=CARTESIAN_POINT('Ctrl Pts',(16.7818328065524,0.,3.98512327200762));
#3839=CARTESIAN_POINT('Ctrl Pts',(18.0021442434375,0.,3.42330192479396));
#3840=CARTESIAN_POINT('Ctrl Pts',(19.1270049692968,0.,3.45147463333956));
#3841=CARTESIAN_POINT('Ctrl Pts',(21.1106762553254,0.,2.59215126849901));
#3842=CARTESIAN_POINT('Ctrl Pts',(24.1154409179203,0.,2.13122905062585));
#3843=CARTESIAN_POINT('Ctrl Pts',(28.7570716465227,0.,2.48541219309353));
#3844=CARTESIAN_POINT('Ctrl Pts',(30.8610725977064,0.,-4.32380575261494));
#3845=CARTESIAN_POINT('Ctrl Pts',(29.2519383950227,0.,-4.77245355836028));
#3846=CARTESIAN_POINT('',(29.2519383950227,1.5,-4.77245355836028));
#3847=CARTESIAN_POINT('Ctrl Pts',(29.2519383950227,1.5,-4.77245355836028));
#3848=CARTESIAN_POINT('Ctrl Pts',(29.2519383950227,-0.660000000000001,-4.77245355836028));
#3849=CARTESIAN_POINT('Ctrl Pts',(21.9641071366747,1.5,-6.80439688368832));
#3850=CARTESIAN_POINT('Ctrl Pts',(21.9641071366747,-0.660000000000001,-6.80439688368832));
#3851=CARTESIAN_POINT('Ctrl Pts',(23.672101274549,1.5,-2.84729812934541));
#3852=CARTESIAN_POINT('Ctrl Pts',(23.672101274549,-0.660000000000001,-2.84729812934541));
#3853=CARTESIAN_POINT('Ctrl Pts',(19.1613411950016,1.5,-3.33371436884934));
#3854=CARTESIAN_POINT('Ctrl Pts',(19.1613411950016,-0.660000000000001,-3.33371436884934));
#3855=CARTESIAN_POINT('Ctrl Pts',(17.2345397051744,1.5,-3.38352975816413));
#3856=CARTESIAN_POINT('Ctrl Pts',(17.2345397051744,-0.660000000000001,-3.38352975816413));
#3857=CARTESIAN_POINT('Ctrl Pts',(16.8377109321552,1.5,-5.12600200141825));
#3858=CARTESIAN_POINT('Ctrl Pts',(16.8377109321552,-0.660000000000001,-5.12600200141825));
#3859=CARTESIAN_POINT('',(16.8377109321552,0.,-5.12600200141825));
#3860=CARTESIAN_POINT('Ctrl Pts',(29.2519383950227,0.,-4.77245355836028));
#3861=CARTESIAN_POINT('Ctrl Pts',(21.9641071366747,0.,-6.80439688368832));
#3862=CARTESIAN_POINT('Ctrl Pts',(23.672101274549,0.,-2.84729812934541));
#3863=CARTESIAN_POINT('Ctrl Pts',(19.1613411950016,0.,-3.33371436884934));
#3864=CARTESIAN_POINT('Ctrl Pts',(17.2345397051744,0.,-3.38352975816413));
#3865=CARTESIAN_POINT('Ctrl Pts',(16.8377109321552,0.,-5.12600200141825));
#3866=CARTESIAN_POINT('',(16.8377109321552,1.5,-5.12600200141825));
#3867=CARTESIAN_POINT('',(16.8377109321552,1.5,-5.12600200141825));
#3868=CARTESIAN_POINT('Ctrl Pts',(29.2519383950227,1.5,-4.77245355836028));
#3869=CARTESIAN_POINT('Ctrl Pts',(21.9641071366747,1.5,-6.80439688368832));
#3870=CARTESIAN_POINT('Ctrl Pts',(23.672101274549,1.5,-2.84729812934541));
#3871=CARTESIAN_POINT('Ctrl Pts',(19.1613411950016,1.5,-3.33371436884934));
#3872=CARTESIAN_POINT('Ctrl Pts',(17.2345397051744,1.5,-3.38352975816413));
#3873=CARTESIAN_POINT('Ctrl Pts',(16.8377109321552,1.5,-5.12600200141825));
#3874=CARTESIAN_POINT('Ctrl Pts',(16.8377109321552,1.5,-5.12600200141825));
#3875=CARTESIAN_POINT('Ctrl Pts',(16.8377109321552,-0.660000000000001,-5.12600200141825));
#3876=CARTESIAN_POINT('Ctrl Pts',(15.1463411250383,1.5,-5.12119887067394));
#3877=CARTESIAN_POINT('Ctrl Pts',(15.1463411250383,-0.660000000000001,-5.12119887067394));
#3878=CARTESIAN_POINT('Ctrl Pts',(6.1690825674038,1.5,-5.20039638916375));
#3879=CARTESIAN_POINT('Ctrl Pts',(6.1690825674038,-0.660000000000001,-5.20039638916375));
#3880=CARTESIAN_POINT('Ctrl Pts',(-6.52362749092467,1.5,-5.5794658499804));
#3881=CARTESIAN_POINT('Ctrl Pts',(-6.52362749092467,-0.660000000000001,
-5.5794658499804));
#3882=CARTESIAN_POINT('Ctrl Pts',(-21.242818604027,1.5,-3.2191168533087));
#3883=CARTESIAN_POINT('Ctrl Pts',(-21.242818604027,-0.660000000000001,-3.2191168533087));
#3884=CARTESIAN_POINT('Ctrl Pts',(-28.1355316629927,1.5,0.120711630909182));
#3885=CARTESIAN_POINT('Ctrl Pts',(-28.1355316629927,-0.660000000000001,
0.120711630909182));
#3886=CARTESIAN_POINT('Ctrl Pts',(-31.0084166862739,1.5,2.67704093130204));
#3887=CARTESIAN_POINT('Ctrl Pts',(-31.0084166862739,-0.660000000000001,
2.67704093130204));
#3888=CARTESIAN_POINT('',(-30.2375369505402,1.5,2.02338898805065));
#3889=CARTESIAN_POINT('Ctrl Pts',(-31.0084164341763,0.49999948762028,2.67704070698238));
#3890=CARTESIAN_POINT('Ctrl Pts',(-30.8800361140849,0.670704692054994,2.5628062839063));
#3891=CARTESIAN_POINT('Ctrl Pts',(-30.7501472100187,0.84126783374662,2.45005907949001));
#3892=CARTESIAN_POINT('Ctrl Pts',(-30.6187111854204,1.01168753355088,2.33873890717364));
#3893=CARTESIAN_POINT('Ctrl Pts',(-30.4930248317139,1.1746522209994,2.23228843748564));
#3894=CARTESIAN_POINT('Ctrl Pts',(-30.365955714005,1.3374507451709,2.12717088547044));
#3895=CARTESIAN_POINT('Ctrl Pts',(-30.2375369505402,1.49999999999988,2.02338898805066));
#3896=CARTESIAN_POINT('Ctrl Pts',(16.8377109321552,1.5,-5.12600200141825));
#3897=CARTESIAN_POINT('Ctrl Pts',(15.1463411250383,1.5,-5.12119887067394));
#3898=CARTESIAN_POINT('Ctrl Pts',(6.1690825674038,1.5,-5.20039638916375));
#3899=CARTESIAN_POINT('Ctrl Pts',(-6.52362749092467,1.5,-5.5794658499804));
#3900=CARTESIAN_POINT('Ctrl Pts',(-20.9096607974693,1.5,-3.27254157538747));
#3901=CARTESIAN_POINT('Ctrl Pts',(-27.5202011308398,1.5,-0.172631746664609));
#3902=CARTESIAN_POINT('Ctrl Pts',(-30.2375369505402,1.5,2.02338898805065));
#3903=CARTESIAN_POINT('Ctrl Pts',(16.8377109321552,0.,-5.12600200141825));
#3904=CARTESIAN_POINT('Ctrl Pts',(15.1463411250383,0.,-5.12119887067394));
#3905=CARTESIAN_POINT('Ctrl Pts',(6.1690825674038,0.,-5.20039638916375));
#3906=CARTESIAN_POINT('Ctrl Pts',(-6.52362749092467,0.,-5.5794658499804));
#3907=CARTESIAN_POINT('Ctrl Pts',(-21.242818604027,0.,-3.2191168533087));
#3908=CARTESIAN_POINT('Ctrl Pts',(-28.1355316629927,0.,0.120711630909182));
#3909=CARTESIAN_POINT('Ctrl Pts',(-31.0084166862739,0.,2.67704093130204));
#3910=CARTESIAN_POINT('Origin',(1.14001967775083,1.5,4.86953436266123));
#3911=CARTESIAN_POINT('Ctrl Pts',(-30.2375369505396,1.49999999999999,2.02338898805013));
#3912=CARTESIAN_POINT('Ctrl Pts',(-30.2337952937897,1.5,2.02663560506344));
#3913=CARTESIAN_POINT('Ctrl Pts',(-30.2300593114649,1.49999999999999,2.02987242063508));
#3914=CARTESIAN_POINT('Ctrl Pts',(-30.2263138882049,1.49999999999999,2.03311253419974));
#3915=CARTESIAN_POINT('Ctrl Pts',(-30.041154668158,1.5,2.19329119995915));
#3916=CARTESIAN_POINT('Ctrl Pts',(-29.8513770723735,1.5,2.34550564113484));
#3917=CARTESIAN_POINT('Ctrl Pts',(-29.657068221066,1.5,2.49017675125092));
#3918=CARTESIAN_POINT('Ctrl Pts',(-29.4583612110577,1.49999999999999,2.63812247545394));
#3919=CARTESIAN_POINT('Ctrl Pts',(-29.2549154411805,1.49999999999999,2.77817943619801));
#3920=CARTESIAN_POINT('Ctrl Pts',(-29.0467943701774,1.49999999999999,2.91075212946208));
#3921=CARTESIAN_POINT('Ctrl Pts',(-28.985856418609,1.49999999999999,2.94956947901001));
#3922=CARTESIAN_POINT('Ctrl Pts',(-28.9245174562325,1.49999999999999,2.98774489874847));
#3923=CARTESIAN_POINT('Ctrl Pts',(-28.8627786201048,1.49999999999999,3.02528784234612));
#3924=CARTESIAN_POINT('Ctrl Pts',(-28.6690138779599,1.5,3.14311479280097));
#3925=CARTESIAN_POINT('Ctrl Pts',(-28.4710912906731,1.5,3.2548427970323));
#3926=CARTESIAN_POINT('Ctrl Pts',(-28.2693705204535,1.50000000000001,3.36065011064977));
#3927=CARTESIAN_POINT('Ctrl Pts',(-28.0602323419797,1.50000000000001,3.47034803027932));
#3928=CARTESIAN_POINT('Ctrl Pts',(-27.8470115970563,1.50000000000001,3.57368195430876));
#3929=CARTESIAN_POINT('Ctrl Pts',(-27.6301398763865,1.50000000000001,3.67089779862402));
#3930=CARTESIAN_POINT('Ctrl Pts',(-27.5380872989039,1.50000000000001,3.71216168039577));
#3931=CARTESIAN_POINT('Ctrl Pts',(-27.4453773123288,1.50000000000001,3.75232386587394));
#3932=CARTESIAN_POINT('Ctrl Pts',(-27.3520444442256,1.50000000000001,3.79140549983965));
#3933=CARTESIAN_POINT('Ctrl Pts',(-27.2326814421543,1.50000000000001,3.84138683279133));
#3934=CARTESIAN_POINT('Ctrl Pts',(-27.1125178794357,1.50000000000001,3.88949706274));
#3935=CARTESIAN_POINT('Ctrl Pts',(-26.9916583952716,1.5,3.93583843065075));
#3936=CARTESIAN_POINT('Ctrl Pts',(-26.8677028427576,1.5,3.98336692957956));
#3937=CARTESIAN_POINT('Ctrl Pts',(-26.7430131862653,1.5,4.0290352724924));
#3938=CARTESIAN_POINT('Ctrl Pts',(-26.6176845498461,1.5,4.07290501477839));
#3939=CARTESIAN_POINT('Ctrl Pts',(-26.5953628406859,1.49999999999999,4.08071845356));
#3940=CARTESIAN_POINT('Ctrl Pts',(-26.5730208653792,1.49999999999999,4.08847470468391));
#3941=CARTESIAN_POINT('Ctrl Pts',(-26.550659184495,1.49999999999999,4.09617393974249));
#3942=CARTESIAN_POINT('Ctrl Pts',(-26.3659847005078,1.49999999999999,4.15975825922633));
#3943=CARTESIAN_POINT('Ctrl Pts',(-26.179975006428,1.49999999999999,4.21950176210725));
#3944=CARTESIAN_POINT('Ctrl Pts',(-25.9929624158959,1.49999999999999,4.27567815256462));
#3945=CARTESIAN_POINT('Ctrl Pts',(-25.9080537125835,1.49999999999999,4.30118373193193));
#3946=CARTESIAN_POINT('Ctrl Pts',(-25.8229384188662,1.49999999999999,4.32595472533356));
#3947=CARTESIAN_POINT('Ctrl Pts',(-25.7376483120083,1.49999999999999,4.35002014717083));
#3948=CARTESIAN_POINT('Ctrl Pts',(-25.5174667344811,1.5,4.41214649147025));
#3949=CARTESIAN_POINT('Ctrl Pts',(-25.2956862586475,1.5,4.4697686002656));
#3950=CARTESIAN_POINT('Ctrl Pts',(-25.0726272188845,1.5,4.52327325815951));
#3951=CARTESIAN_POINT('Ctrl Pts',(-24.830594648481,1.5,4.58132905312924));
#3952=CARTESIAN_POINT('Ctrl Pts',(-24.587056772788,1.5,4.63453724241089));
#3953=CARTESIAN_POINT('Ctrl Pts',(-24.342435232932,1.5,4.68345442597066));
#3954=CARTESIAN_POINT('Ctrl Pts',(-24.0806904412321,1.5,4.73579576119788));
#3955=CARTESIAN_POINT('Ctrl Pts',(-23.8177051001542,1.5,4.78322501460086));
#3956=CARTESIAN_POINT('Ctrl Pts',(-23.554008139782,1.5,4.82648647475461));
#3957=CARTESIAN_POINT('Ctrl Pts',(-23.2405244203756,1.5,4.87791582538803));
#3958=CARTESIAN_POINT('Ctrl Pts',(-22.92603517214,1.5,4.9234558821029));
#3959=CARTESIAN_POINT('Ctrl Pts',(-22.6114439723032,1.5,4.96443227490802));
#3960=CARTESIAN_POINT('Ctrl Pts',(-22.5446347761331,1.5,4.97313436151018));
#3961=CARTESIAN_POINT('Ctrl Pts',(-22.4778210194986,1.5,4.9816308147111));
#3962=CARTESIAN_POINT('Ctrl Pts',(-22.4110114057897,1.5,4.98993457808753));
#3963=CARTESIAN_POINT('Ctrl Pts',(-22.1508063610361,1.50000000000001,5.02227544942385));
#3964=CARTESIAN_POINT('Ctrl Pts',(-21.8925698598374,1.5,5.05138331788897));
#3965=CARTESIAN_POINT('Ctrl Pts',(-21.6386197859862,1.5,5.07781979513669));
#3966=CARTESIAN_POINT('Ctrl Pts',(-21.3769007661508,1.5,5.10506502806082));
#3967=CARTESIAN_POINT('Ctrl Pts',(-21.1197360819527,1.5,5.12947999537432));
#3968=CARTESIAN_POINT('Ctrl Pts',(-20.8696606678661,1.5,5.15169330709646));
#3969=CARTESIAN_POINT('Ctrl Pts',(-20.8191072598628,1.5,5.15618378695709));
#3970=CARTESIAN_POINT('Ctrl Pts',(-20.7688435066458,1.5,5.16058413868542));
#3971=CARTESIAN_POINT('Ctrl Pts',(-20.7188902492778,1.5,5.16489923127004));
#3972=CARTESIAN_POINT('Ctrl Pts',(-20.5041147969358,1.5,5.18345209469855));
#3973=CARTESIAN_POINT('Ctrl Pts',(-20.2950635510776,1.5,5.20034230108586));
#3974=CARTESIAN_POINT('Ctrl Pts',(-20.0933847656336,1.5,5.21564597030981));
#3975=CARTESIAN_POINT('Ctrl Pts',(-19.8715555619165,1.5,5.23247868154627));
#3976=CARTESIAN_POINT('Ctrl Pts',(-19.6586456330018,1.5,5.24739212952468));
#3977=CARTESIAN_POINT('Ctrl Pts',(-19.4568491468652,1.5,5.26055530564244));
#3978=CARTESIAN_POINT('Ctrl Pts',(-19.3049736457191,1.5,5.2704621380548));
#3979=CARTESIAN_POINT('Ctrl Pts',(-19.1593931820414,1.5,5.27937921742333));
#3980=CARTESIAN_POINT('Ctrl Pts',(-19.0210433870338,1.5,5.28739765571153));
#3981=CARTESIAN_POINT('Ctrl Pts',(-18.9711489355537,1.5,5.29028942421827));
#3982=CARTESIAN_POINT('Ctrl Pts',(-18.9221953644963,1.5,5.29306443545563));
#3983=CARTESIAN_POINT('Ctrl Pts',(-18.8742268000768,1.5,5.29572728213782));
#3984=CARTESIAN_POINT('Ctrl Pts',(-18.864824040027,1.5,5.29624925123789));
#3985=CARTESIAN_POINT('Ctrl Pts',(-18.8554560953261,1.5,5.2967670756345));
#3986=CARTESIAN_POINT('Ctrl Pts',(-18.8461471198503,1.5,5.29727948613276));
#3987=CARTESIAN_POINT('Ctrl Pts',(-18.7334862426067,1.5,5.3034808792284));
#3988=CARTESIAN_POINT('Ctrl Pts',(-18.6287310561587,1.5,5.30893490230097));
#3989=CARTESIAN_POINT('Ctrl Pts',(-18.5299112214963,1.5,5.31385439992691));
#3990=CARTESIAN_POINT('Ctrl Pts',(-18.4256380647603,1.5,5.31904537751521));
#3991=CARTESIAN_POINT('Ctrl Pts',(-18.3279734082384,1.5,5.32364078378197));
#3992=CARTESIAN_POINT('Ctrl Pts',(-18.2346016229507,1.5,5.32783073841533));
#3993=CARTESIAN_POINT('Ctrl Pts',(-18.1369546918885,1.5,5.33221253544296));
#3994=CARTESIAN_POINT('Ctrl Pts',(-18.0440027361324,1.5,5.33615054430275));
#3995=CARTESIAN_POINT('Ctrl Pts',(-17.9530965415633,1.5,5.33980494028624));
#3996=CARTESIAN_POINT('Ctrl Pts',(-17.9025040122938,1.5,5.34183874157595));
#3997=CARTESIAN_POINT('Ctrl Pts',(-17.8525451081636,1.5,5.34378373847719));
#3998=CARTESIAN_POINT('Ctrl Pts',(-17.8027630804267,1.5,5.34566078906948));
#3999=CARTESIAN_POINT('Ctrl Pts',(-17.7855305147468,1.5,5.34631054961735));
#4000=CARTESIAN_POINT('Ctrl Pts',(-17.7683191431228,1.5,5.34695212794483));
#4001=CARTESIAN_POINT('Ctrl Pts',(-17.7511100182894,1.5,5.34758626185815));
#4002=CARTESIAN_POINT('Ctrl Pts',(-17.7336280300427,1.5,5.34823045043408));
#4003=CARTESIAN_POINT('Ctrl Pts',(-17.7161523646819,1.5,5.34886680123599));
#4004=CARTESIAN_POINT('Ctrl Pts',(-17.6986908876287,1.5,5.3494950560435));
#4005=CARTESIAN_POINT('Ctrl Pts',(-17.3035641688426,1.5,5.36371150863198));
#4006=CARTESIAN_POINT('Ctrl Pts',(-16.9144695187083,1.5,5.37383244203566));
#4007=CARTESIAN_POINT('Ctrl Pts',(-16.5308798263576,1.5,5.3802221035256));
#4008=CARTESIAN_POINT('Ctrl Pts',(-16.2250165106129,1.5,5.38531703461675));
#4009=CARTESIAN_POINT('Ctrl Pts',(-15.922653236192,1.5,5.38803851156023));
#4010=CARTESIAN_POINT('Ctrl Pts',(-15.6235224734428,1.5,5.38854751646289));
#4011=CARTESIAN_POINT('Ctrl Pts',(-15.2342893805637,1.5,5.38920984069437));
#4012=CARTESIAN_POINT('Ctrl Pts',(-14.8505224896553,1.5,5.38612774065209));
#4013=CARTESIAN_POINT('Ctrl Pts',(-14.4716416695502,1.5,5.37959707331161));
#4014=CARTESIAN_POINT('Ctrl Pts',(-14.0859965104277,1.5,5.37294981086904));
#4015=CARTESIAN_POINT('Ctrl Pts',(-13.7054134455504,1.5,5.36272969242992));
#4016=CARTESIAN_POINT('Ctrl Pts',(-13.3292800193233,1.5,5.34919404558174));
#4017=CARTESIAN_POINT('Ctrl Pts',(-12.9565439992755,1.5,5.33578065878022));
#4018=CARTESIAN_POINT('Ctrl Pts',(-12.5881775953025,1.5,5.31911110583216));
#4019=CARTESIAN_POINT('Ctrl Pts',(-12.2235841570957,1.5,5.29938532633141));
#4020=CARTESIAN_POINT('Ctrl Pts',(-11.9125827069805,1.5,5.28255906072566));
#4021=CARTESIAN_POINT('Ctrl Pts',(-11.6043350479086,1.5,5.26343720653592));
#4022=CARTESIAN_POINT('Ctrl Pts',(-11.2984729831696,1.5,5.2423417983655));
#4023=CARTESIAN_POINT('Ctrl Pts',(-11.0387538851364,1.5,5.22442888593114));
#4024=CARTESIAN_POINT('Ctrl Pts',(-10.7807545217096,1.5,5.20509175026844));
#4025=CARTESIAN_POINT('Ctrl Pts',(-10.5242437369439,1.5,5.18449881210053));
#4026=CARTESIAN_POINT('Ctrl Pts',(-10.1804515117854,1.5,5.15689883402645));
#4027=CARTESIAN_POINT('Ctrl Pts',(-9.83933390510173,1.5,5.12707624458748));
#4028=CARTESIAN_POINT('Ctrl Pts',(-9.50033155741444,1.5,5.0954487571781));
#4029=CARTESIAN_POINT('Ctrl Pts',(-9.27567015075047,1.5,5.07448879669666));
#4030=CARTESIAN_POINT('Ctrl Pts',(-9.05193787862125,1.5,5.05273488616363));
#4031=CARTESIAN_POINT('Ctrl Pts',(-8.82897326682209,1.5,5.03029627520487));
#4032=CARTESIAN_POINT('Ctrl Pts',(-8.44288843028761,1.5,4.99144164543124));
#4033=CARTESIAN_POINT('Ctrl Pts',(-8.05910111634218,1.5,4.95055906622723));
#4034=CARTESIAN_POINT('Ctrl Pts',(-7.67677701721786,1.5,4.90814164011349));
#4035=CARTESIAN_POINT('Ctrl Pts',(-7.4041297573418,1.5,4.87789244832203));
#4036=CARTESIAN_POINT('Ctrl Pts',(-7.13222678735648,1.5,4.84686119117315));
#4037=CARTESIAN_POINT('Ctrl Pts',(-6.86076721285879,1.5,4.81521112359619));
#4038=CARTESIAN_POINT('Ctrl Pts',(-6.8229722811227,1.5,4.8108045295546));
#4039=CARTESIAN_POINT('Ctrl Pts',(-6.78518594616242,1.5,4.80638592407432));
#4040=CARTESIAN_POINT('Ctrl Pts',(-6.7474073974805,1.5,4.80195573309565));
#4041=CARTESIAN_POINT('Ctrl Pts',(-6.73441476210259,1.5,4.80043212093879));
#4042=CARTESIAN_POINT('Ctrl Pts',(-6.72141925548236,1.5,4.79890669429121));
#4043=CARTESIAN_POINT('Ctrl Pts',(-6.70841347214424,1.5,4.79737859996483));
#4044=CARTESIAN_POINT('Ctrl Pts',(-6.48267459125147,1.5,4.770855760535));
#4045=CARTESIAN_POINT('Ctrl Pts',(-6.25456998290655,1.5,4.74361006590382));
#4046=CARTESIAN_POINT('Ctrl Pts',(-6.02781808108521,1.5,4.71618895197073));
#4047=CARTESIAN_POINT('Ctrl Pts',(-5.61980678153037,1.5,4.6668481339171));
#4048=CARTESIAN_POINT('Ctrl Pts',(-5.21617467425362,1.5,4.61694421711996));
#4049=CARTESIAN_POINT('Ctrl Pts',(-4.83856112378684,1.5,4.5698878566956));
#4050=CARTESIAN_POINT('Ctrl Pts',(-4.6969560423618,1.5,4.55224172153646));
#4051=CARTESIAN_POINT('Ctrl Pts',(-4.55900979339634,1.5,4.53499627493262));
#4052=CARTESIAN_POINT('Ctrl Pts',(-4.42586408354591,1.5,4.51832611180184));
#4053=CARTESIAN_POINT('Ctrl Pts',(-4.40427308746376,1.5,4.51562286715919));
#4054=CARTESIAN_POINT('Ctrl Pts',(-4.38280832834808,1.5,4.51293473531525));
#4055=CARTESIAN_POINT('Ctrl Pts',(-4.36147467664027,1.5,4.51026244236388));
#4056=CARTESIAN_POINT('Ctrl Pts',(-4.34931105189763,1.5,4.50873880407129));
#4057=CARTESIAN_POINT('Ctrl Pts',(-4.33719246839501,1.5,4.50722061789631));
#4058=CARTESIAN_POINT('Ctrl Pts',(-4.32511184432304,1.5,4.50570701714359));
#4059=CARTESIAN_POINT('Ctrl Pts',(-4.10118642391084,1.5,4.47765104231391));
#4060=CARTESIAN_POINT('Ctrl Pts',(-3.88867243419537,1.5,4.45097091827309));
#4061=CARTESIAN_POINT('Ctrl Pts',(-3.68522030236831,1.5,4.42546582810022));
#4062=CARTESIAN_POINT('Ctrl Pts',(-3.42827353994682,1.5,4.39325456402381));
#4063=CARTESIAN_POINT('Ctrl Pts',(-3.1857805977361,1.5,4.36291637676583));
#4064=CARTESIAN_POINT('Ctrl Pts',(-2.95301755734803,1.5,4.33396311712648));
#4065=CARTESIAN_POINT('Ctrl Pts',(-2.64467597250301,1.5,4.2956086861621));
#4066=CARTESIAN_POINT('Ctrl Pts',(-2.35340950786154,1.5,4.2596775987671));
#4067=CARTESIAN_POINT('Ctrl Pts',(-2.06824404682498,1.5,4.22496787940098));
#4068=CARTESIAN_POINT('Ctrl Pts',(-1.8533186349837,1.5,4.19880762597287));
#4069=CARTESIAN_POINT('Ctrl Pts',(-1.64186374211442,1.5,4.1733370064896));
#4070=CARTESIAN_POINT('Ctrl Pts',(-1.42916964311695,1.5,4.14805861485451));
#4071=CARTESIAN_POINT('Ctrl Pts',(-1.24078810701873,1.5,4.12566973679558));
#4072=CARTESIAN_POINT('Ctrl Pts',(-1.05143453978735,1.5,4.10343097364107));
#4073=CARTESIAN_POINT('Ctrl Pts',(-0.857832534542974,1.5,4.08103919940624));
#4074=CARTESIAN_POINT('Ctrl Pts',(-0.68880652471363,1.5,4.06148985513608));
#4075=CARTESIAN_POINT('Ctrl Pts',(-0.51654223225136,1.5,4.04182373011371));
#4076=CARTESIAN_POINT('Ctrl Pts',(-0.338855474791857,1.5,4.02187807261217));
#4077=CARTESIAN_POINT('Ctrl Pts',(-0.172282687709815,1.5,4.00317997823689));
#4078=CARTESIAN_POINT('Ctrl Pts',(-0.000944601626649944,1.5,3.98423570945314));
#4079=CARTESIAN_POINT('Ctrl Pts',(0.176962309038757,1.5,3.96495299846918));
#4080=CARTESIAN_POINT('Ctrl Pts',(0.351606668284712,1.5,3.94602390408086));
#4081=CARTESIAN_POINT('Ctrl Pts',(0.532581040071602,1.5,3.92676768274042));
#4082=CARTESIAN_POINT('Ctrl Pts',(0.72159670751355,1.5,3.90714994018427));
#4083=CARTESIAN_POINT('Ctrl Pts',(0.889047570336262,1.5,3.8897703866154));
#4084=CARTESIAN_POINT('Ctrl Pts',(1.06280953667672,1.5,3.87210711157171));
#4085=CARTESIAN_POINT('Ctrl Pts',(1.24407702413679,1.5,3.8541829909191));
#4086=CARTESIAN_POINT('Ctrl Pts',(1.26742117348904,1.5,3.85187467101361));
#4087=CARTESIAN_POINT('Ctrl Pts',(1.29088980907388,1.5,3.84956209597365));
#4088=CARTESIAN_POINT('Ctrl Pts',(1.31448548841964,1.5,3.8472453802817));
#4089=CARTESIAN_POINT('Ctrl Pts',(1.42899700200292,1.5,3.83600219391104));
#4090=CARTESIAN_POINT('Ctrl Pts',(1.54649813261794,1.5,3.82464411253794));
#4091=CARTESIAN_POINT('Ctrl Pts',(1.6672770820639,1.5,3.81314819462295));
#4092=CARTESIAN_POINT('Ctrl Pts',(1.68548104283269,1.5,3.81141551488294));
#4093=CARTESIAN_POINT('Ctrl Pts',(1.70375400162177,1.5,3.80968021475685));
#4094=CARTESIAN_POINT('Ctrl Pts',(1.72212820038232,1.5,3.80793925503593));
#4095=CARTESIAN_POINT('Ctrl Pts',(1.8950448493804,1.5,3.79155536124524));
#4096=CARTESIAN_POINT('Ctrl Pts',(2.07645857851809,1.5,3.77471937250263));
#4097=CARTESIAN_POINT('Ctrl Pts',(2.26533613202404,1.5,3.75753239704228));
#4098=CARTESIAN_POINT('Ctrl Pts',(2.45451985028614,1.5,3.74031756201867));
#4099=CARTESIAN_POINT('Ctrl Pts',(2.65119161904104,1.5,3.7227506958672));
#4100=CARTESIAN_POINT('Ctrl Pts',(2.85430796830265,1.5,3.7048805235274));
#4101=CARTESIAN_POINT('Ctrl Pts',(3.06086450365666,1.5,3.68670768368409));
#4102=CARTESIAN_POINT('Ctrl Pts',(3.27408576401215,1.5,3.66822109255634));
#4103=CARTESIAN_POINT('Ctrl Pts',(3.49286897045564,1.5,3.6494170293364));
#4104=CARTESIAN_POINT('Ctrl Pts',(3.72558179917576,1.5,3.62941573758061));
#4105=CARTESIAN_POINT('Ctrl Pts',(3.96458735551702,1.5,3.60905518307288));
#4106=CARTESIAN_POINT('Ctrl Pts',(4.20855252728194,1.5,3.58826965400713));
#4107=CARTESIAN_POINT('Ctrl Pts',(4.37184747684828,1.5,3.57435712749383));
#4108=CARTESIAN_POINT('Ctrl Pts',(4.53736426395281,1.5,3.56025287349266));
#4109=CARTESIAN_POINT('Ctrl Pts',(4.70470187755637,1.5,3.54592444027639));
#4110=CARTESIAN_POINT('Ctrl Pts',(4.98380030472694,1.5,3.52202638718263));
#4111=CARTESIAN_POINT('Ctrl Pts',(5.26774502017556,1.5,3.49754691833425));
#4112=CARTESIAN_POINT('Ctrl Pts',(5.55524949715075,1.5,3.47220567087764));
#4113=CARTESIAN_POINT('Ctrl Pts',(5.93341654493371,1.5,3.43887323432351));
#4114=CARTESIAN_POINT('Ctrl Pts',(6.31774234964862,1.5,3.40404822381377));
#4115=CARTESIAN_POINT('Ctrl Pts',(6.70527769826349,1.5,3.36700056442672));
#4116=CARTESIAN_POINT('Ctrl Pts',(7.04422598225608,1.5,3.33459773815535));
#4117=CARTESIAN_POINT('Ctrl Pts',(7.38562841725574,1.5,3.30048928723064));
#4118=CARTESIAN_POINT('Ctrl Pts',(7.72750891122856,1.5,3.26419008408891));
#4119=CARTESIAN_POINT('Ctrl Pts',(7.84926141411927,1.5,3.25126299724611));
#4120=CARTESIAN_POINT('Ctrl Pts',(7.97107458551754,1.5,3.23805844494137));
#4121=CARTESIAN_POINT('Ctrl Pts',(8.09285941000345,1.5,3.22455637168536));
#4122=CARTESIAN_POINT('Ctrl Pts',(8.37921768375685,1.5,3.19280832420898));
#4123=CARTESIAN_POINT('Ctrl Pts',(8.66543795848237,1.5,3.15943873922727));
#4124=CARTESIAN_POINT('Ctrl Pts',(8.95033395522809,1.5,3.12409127077656));
#4125=CARTESIAN_POINT('Ctrl Pts',(9.18845852070908,1.5,3.09454680310476));
#4126=CARTESIAN_POINT('Ctrl Pts',(9.42565794543148,1.5,3.06362062240277));
#4127=CARTESIAN_POINT('Ctrl Pts',(9.66124991551543,1.5,3.03114544574892));
#4128=CARTESIAN_POINT('Ctrl Pts',(9.886670020665,1.5,3.00007240988334));
#4129=CARTESIAN_POINT('Ctrl Pts',(10.1106183714759,1.5,2.96758081885689));
#4130=CARTESIAN_POINT('Ctrl Pts',(10.3325085538622,1.5,2.93356848320867));
#4131=CARTESIAN_POINT('Ctrl Pts',(10.5440562437169,1.5,2.90114149182236));
#4132=CARTESIAN_POINT('Ctrl Pts',(10.753733117056,1.5,2.86733205096079));
#4133=CARTESIAN_POINT('Ctrl Pts',(10.9610425166206,1.5,2.83209688558433));
#4134=CARTESIAN_POINT('Ctrl Pts',(11.1247121753544,1.5,2.80427891155754));
#4135=CARTESIAN_POINT('Ctrl Pts',(11.2869063881666,1.5,2.77557308549288));
#4136=CARTESIAN_POINT('Ctrl Pts',(11.4473864461662,1.5,2.74598048905742));
#4137=CARTESIAN_POINT('Ctrl Pts',(11.553597493978,1.5,2.72639512303711));
#4138=CARTESIAN_POINT('Ctrl Pts',(11.6591804005066,1.5,2.70647589362988));
#4139=CARTESIAN_POINT('Ctrl Pts',(11.76367159676,1.5,2.68594799574105));
#4140=CARTESIAN_POINT('Ctrl Pts',(11.7964550844154,1.5,2.67950749059649));
#4141=CARTESIAN_POINT('Ctrl Pts',(11.829131199191,1.5,2.67300742457918));
#4142=CARTESIAN_POINT('Ctrl Pts',(11.8616859025202,1.5,2.6664404037272));
#4143=CARTESIAN_POINT('Ctrl Pts',(12.0008154873567,1.5,2.63837481592222));
#4144=CARTESIAN_POINT('Ctrl Pts',(12.1378233663548,1.49999999999999,2.6089918119749));
#4145=CARTESIAN_POINT('Ctrl Pts',(12.2734880318177,1.5,2.57708405230406));
#4146=CARTESIAN_POINT('Ctrl Pts',(12.3720491713233,1.5,2.55390288614339));
#4147=CARTESIAN_POINT('Ctrl Pts',(12.4698925440469,1.5,2.52935494370487));
#4148=CARTESIAN_POINT('Ctrl Pts',(12.5673303176919,1.5,2.503028111913));
#4149=CARTESIAN_POINT('Ctrl Pts',(12.6536663943788,1.5,2.47970086126389));
#4150=CARTESIAN_POINT('Ctrl Pts',(12.7396841195956,1.5,2.45497733455598));
#4151=CARTESIAN_POINT('Ctrl Pts',(12.8255910274147,1.5,2.42853300000139));
#4152=CARTESIAN_POINT('Ctrl Pts',(12.9114979352338,1.5,2.40208866544679));
#4153=CARTESIAN_POINT('Ctrl Pts',(12.9972942860165,1.5,2.37392454644978));
#4154=CARTESIAN_POINT('Ctrl Pts',(13.0831746516526,1.5,2.34366516065363));
#4155=CARTESIAN_POINT('Ctrl Pts',(13.1659810649101,1.5,2.31448886189672));
#4156=CARTESIAN_POINT('Ctrl Pts',(13.248863365756,1.5,2.28335555594758));
#4157=CARTESIAN_POINT('Ctrl Pts',(13.3320214711795,1.5,2.25002943668965));
#4158=CARTESIAN_POINT('Ctrl Pts',(13.4134355307938,1.5,2.2174022544546));
#4159=CARTESIAN_POINT('Ctrl Pts',(13.4951139958824,1.50000000000001,2.18267346241825));
#4160=CARTESIAN_POINT('Ctrl Pts',(13.5772322422152,1.50000000000001,2.14557372974471));
#4161=CARTESIAN_POINT('Ctrl Pts',(13.6568886107536,1.50000000000001,2.10958623475434));
#4162=CARTESIAN_POINT('Ctrl Pts',(13.7369588186311,1.50000000000001,2.07136795327505));
#4163=CARTESIAN_POINT('Ctrl Pts',(13.8175907589904,1.50000000000001,2.03062519205916));
#4164=CARTESIAN_POINT('Ctrl Pts',(13.8337964027114,1.50000000000001,2.02243659248517));
#4165=CARTESIAN_POINT('Ctrl Pts',(13.8500246957313,1.50000000000001,2.014145855992));
#4166=CARTESIAN_POINT('Ctrl Pts',(13.8662767749019,1.50000000000001,2.00575034734995));
#4167=CARTESIAN_POINT('Ctrl Pts',(13.9081642812626,1.50000000000001,1.98411207461237));
#4168=CARTESIAN_POINT('Ctrl Pts',(13.950461030891,1.50000000000001,1.96165528000694));
#4169=CARTESIAN_POINT('Ctrl Pts',(13.9926697842201,1.5,1.93862227096309));
#4170=CARTESIAN_POINT('Ctrl Pts',(14.0142784190252,1.5,1.92683059644927));
#4171=CARTESIAN_POINT('Ctrl Pts',(14.0358641984505,1.5,1.91488871790894));
#4172=CARTESIAN_POINT('Ctrl Pts',(14.0573617100153,1.49999999999999,1.90283427700156));
#4173=CARTESIAN_POINT('Ctrl Pts',(14.0897595100142,1.49999999999999,1.88466764574106));
#4174=CARTESIAN_POINT('Ctrl Pts',(14.1213372809979,1.49999999999999,1.86659470623033));
#4175=CARTESIAN_POINT('Ctrl Pts',(14.1521991517948,1.5,1.84860499061564));
#4176=CARTESIAN_POINT('Ctrl Pts',(14.184396915122,1.5,1.82983656891176));
#4177=CARTESIAN_POINT('Ctrl Pts',(14.2158029519234,1.50000000000002,1.81113812163914));
#4178=CARTESIAN_POINT('Ctrl Pts',(14.2465771364748,1.50000000000001,1.79256971204494));
#4179=CARTESIAN_POINT('Ctrl Pts',(14.2814551303541,1.49999999999999,1.77152516169812));
#4180=CARTESIAN_POINT('Ctrl Pts',(14.3155518423707,1.49999999999999,1.75069273316637));
#4181=CARTESIAN_POINT('Ctrl Pts',(14.3491101294543,1.49999999999998,1.73017817585942));
#4182=CARTESIAN_POINT('Ctrl Pts',(14.3779858740141,1.49999999999998,1.71252610931982));
#4183=CARTESIAN_POINT('Ctrl Pts',(14.4064625536128,1.49999999999998,1.69510776450755));
#4184=CARTESIAN_POINT('Ctrl Pts',(14.4346889400213,1.49999999999999,1.67796712650023));
#4185=CARTESIAN_POINT('Ctrl Pts',(14.4984589258247,1.5,1.63924243016231));
#4186=CARTESIAN_POINT('Ctrl Pts',(14.5609266774462,1.49999999999999,1.60191409094533));
#4187=CARTESIAN_POINT('Ctrl Pts',(14.6235034279238,1.49999999999999,1.56612658872582));
#4188=CARTESIAN_POINT('Ctrl Pts',(14.6623030990163,1.49999999999999,1.54393714448749));
#4189=CARTESIAN_POINT('Ctrl Pts',(14.7010798634147,1.49999999999999,1.52237211616235));
#4190=CARTESIAN_POINT('Ctrl Pts',(14.7402377283426,1.49999999999999,1.50142071435942));
#4191=CARTESIAN_POINT('Ctrl Pts',(14.7758873808755,1.49999999999999,1.48234638035967));
#4192=CARTESIAN_POINT('Ctrl Pts',(14.8118524075414,1.49999999999999,1.46377995768135));
#4193=CARTESIAN_POINT('Ctrl Pts',(14.8484505281561,1.49999999999999,1.44575260484134));
#4194=CARTESIAN_POINT('Ctrl Pts',(14.8815568628569,1.49999999999999,1.42944522165149));
#4195=CARTESIAN_POINT('Ctrl Pts',(14.9151810332879,1.49999999999999,1.41357870584738));
#4196=CARTESIAN_POINT('Ctrl Pts',(14.9495737189396,1.5,1.39821557530277));
#4197=CARTESIAN_POINT('Ctrl Pts',(14.9693267160288,1.5,1.38939195867676));
#4198=CARTESIAN_POINT('Ctrl Pts',(14.9893335232394,1.5,1.38073514573342));
#4199=CARTESIAN_POINT('Ctrl Pts',(15.0096447310109,1.5,1.37226431791822));
#4200=CARTESIAN_POINT('Ctrl Pts',(15.0722269561691,1.5,1.34616428193956));
#4201=CARTESIAN_POINT('Ctrl Pts',(15.1378964880444,1.5,1.32173616111247));
#4202=CARTESIAN_POINT('Ctrl Pts',(15.206402740382,1.5,1.30048138533187));
#4203=CARTESIAN_POINT('Ctrl Pts',(15.2573606011224,1.5,1.28467118017042));
#4204=CARTESIAN_POINT('Ctrl Pts',(15.3098890700018,1.5,1.2706197125179));
#4205=CARTESIAN_POINT('Ctrl Pts',(15.3638774142426,1.5,1.2589237086481));
#4206=CARTESIAN_POINT('Ctrl Pts',(15.3824694154108,1.5,1.25489594819965));
#4207=CARTESIAN_POINT('Ctrl Pts',(15.4012344108101,1.5,1.25114715061918));
#4208=CARTESIAN_POINT('Ctrl Pts',(15.4201673421117,1.5,1.24770018911881));
#4209=CARTESIAN_POINT('Ctrl Pts',(15.4480170350895,1.5,1.24262982690376));
#4210=CARTESIAN_POINT('Ctrl Pts',(15.4761145444581,1.5,1.23824102619373));
#4211=CARTESIAN_POINT('Ctrl Pts',(15.5042043297991,1.5,1.23461144646394));
#4212=CARTESIAN_POINT('Ctrl Pts',(15.5318620946041,1.5,1.23103768962352));
#4213=CARTESIAN_POINT('Ctrl Pts',(15.5595122873754,1.5,1.2282001066137));
#4214=CARTESIAN_POINT('Ctrl Pts',(15.5869091734653,1.5,1.2261221612424));
#4215=CARTESIAN_POINT('Ctrl Pts',(15.6142008008716,1.5,1.22405219932561));
#4216=CARTESIAN_POINT('Ctrl Pts',(15.6412409879309,1.5,1.22273610252946));
#4217=CARTESIAN_POINT('Ctrl Pts',(15.6677862089015,1.5,1.22214489863002));
#4218=CARTESIAN_POINT('Ctrl Pts',(15.6945406231681,1.5,1.22154903566623));
#4219=CARTESIAN_POINT('Ctrl Pts',(15.7207921702355,1.5,1.2216894969672));
#4220=CARTESIAN_POINT('Ctrl Pts',(15.7462920004296,1.5,1.22248322281614));
#4221=CARTESIAN_POINT('Ctrl Pts',(15.7726196829026,1.5,1.22330271698386));
#4222=CARTESIAN_POINT('Ctrl Pts',(15.7981459809862,1.5,1.22481849422764));
#4223=CARTESIAN_POINT('Ctrl Pts',(15.8225985815198,1.5,1.22688296680944));
#4224=CARTESIAN_POINT('Ctrl Pts',(15.8316370729344,1.5,1.2276460642837));
#4225=CARTESIAN_POINT('Ctrl Pts',(15.84052888648,1.5,1.22848360035794));
#4226=CARTESIAN_POINT('Ctrl Pts',(15.8492603460339,1.5,1.22938635857439));
#4227=CARTESIAN_POINT('Ctrl Pts',(15.8752106760547,1.5,1.23206940068224));
#4228=CARTESIAN_POINT('Ctrl Pts',(15.9002189981378,1.5,1.23539390779828));
#4229=CARTESIAN_POINT('Ctrl Pts',(15.9242319250192,1.5,1.23919918936648));
#4230=CARTESIAN_POINT('Ctrl Pts',(15.9501886120697,1.5,1.24331249480788));
#4231=CARTESIAN_POINT('Ctrl Pts',(15.974982600101,1.5,1.24798743511524));
#4232=CARTESIAN_POINT('Ctrl Pts',(15.9986007079772,1.5,1.25305595421041));
#4233=CARTESIAN_POINT('Ctrl Pts',(16.0207226927192,1.5,1.25780340064751));
#4234=CARTESIAN_POINT('Ctrl Pts',(16.0418141788407,1.5,1.26289667008938));
#4235=CARTESIAN_POINT('Ctrl Pts',(16.0618970949743,1.5,1.26822275322431));
#4236=CARTESIAN_POINT('Ctrl Pts',(16.0882246094682,1.49999999999999,1.27520493300331));
#4237=CARTESIAN_POINT('Ctrl Pts',(16.1138379307147,1.49999999999999,1.28283870442167));
#4238=CARTESIAN_POINT('Ctrl Pts',(16.1389630519792,1.49999999999999,1.29112215414976));
#4239=CARTESIAN_POINT('Ctrl Pts',(16.1644211208015,1.49999999999999,1.29951537267571));
#4240=CARTESIAN_POINT('Ctrl Pts',(16.1893779380213,1.49999999999999,1.30857567974431));
#4241=CARTESIAN_POINT('Ctrl Pts',(16.2140509832687,1.5,1.31835164075651));
#4242=CARTESIAN_POINT('Ctrl Pts',(16.2308102903248,1.5,1.32499201816954));
#4243=CARTESIAN_POINT('Ctrl Pts',(16.2474383074032,1.5,1.33196362561461));
#4244=CARTESIAN_POINT('Ctrl Pts',(16.2639986895245,1.5,1.33929460616079));
#4245=CARTESIAN_POINT('Ctrl Pts',(16.2925242729341,1.50000000000001,1.35192236411413));
#4246=CARTESIAN_POINT('Ctrl Pts',(16.3205868967279,1.5,1.36552327695976));
#4247=CARTESIAN_POINT('Ctrl Pts',(16.348180133584,1.5,1.38003619580369));
#4248=CARTESIAN_POINT('Ctrl Pts',(16.376380791422,1.5,1.39486859334674));
#4249=CARTESIAN_POINT('Ctrl Pts',(16.4040926941819,1.49999999999999,1.41065437194904));
#4250=CARTESIAN_POINT('Ctrl Pts',(16.4312911408889,1.49999999999999,1.42737762082488));
#4251=CARTESIAN_POINT('Ctrl Pts',(16.4390157188017,1.49999999999999,1.43212715818957));
#4252=CARTESIAN_POINT('Ctrl Pts',(16.4466986927062,1.49999999999999,1.43695257148943));
#4253=CARTESIAN_POINT('Ctrl Pts',(16.4543389695688,1.49999999999999,1.44185406580663));
#4254=CARTESIAN_POINT('Ctrl Pts',(16.4764978585172,1.49999999999999,1.45606973759572));
#4255=CARTESIAN_POINT('Ctrl Pts',(16.4984000805429,1.49999999999999,1.47097635009296));
#4256=CARTESIAN_POINT('Ctrl Pts',(16.5198521810087,1.49999999999999,1.48643402849482));
#4257=CARTESIAN_POINT('Ctrl Pts',(16.5419826698061,1.49999999999999,1.50238053122786));
#4258=CARTESIAN_POINT('Ctrl Pts',(16.5636341493956,1.49999999999999,1.51891346464515));
#4259=CARTESIAN_POINT('Ctrl Pts',(16.5846293319728,1.49999999999999,1.53583491243833));
#4260=CARTESIAN_POINT('Ctrl Pts',(16.5989255129361,1.49999999999999,1.5473571785069));
#4261=CARTESIAN_POINT('Ctrl Pts',(16.6129181448062,1.49999999999999,1.55905863572717));
#4262=CARTESIAN_POINT('Ctrl Pts',(16.6265597698144,1.5,1.57086604116992));
#4263=CARTESIAN_POINT('Ctrl Pts',(16.6572577480919,1.5,1.59743644429841));
#4264=CARTESIAN_POINT('Ctrl Pts',(16.6863334374287,1.5,1.62473096009712));
#4265=CARTESIAN_POINT('Ctrl Pts',(16.7138746062607,1.5,1.65239273695287));
#4266=CARTESIAN_POINT('Ctrl Pts',(16.7417717673141,1.49999999999999,1.68041206498768));
#4267=CARTESIAN_POINT('Ctrl Pts',(16.7680945286679,1.49999999999999,1.70880833035569));
#4268=CARTESIAN_POINT('Ctrl Pts',(16.7929376483549,1.49999999999999,1.73726493227113));
#4269=CARTESIAN_POINT('Ctrl Pts',(16.8183752648702,1.49999999999998,1.76640250178618));
#4270=CARTESIAN_POINT('Ctrl Pts',(16.8422616279212,1.49999999999998,1.7956033909819));
#4271=CARTESIAN_POINT('Ctrl Pts',(16.8647014075051,1.49999999999997,1.82458300822481));
#4272=CARTESIAN_POINT('Ctrl Pts',(16.8820172700989,1.49999999999997,1.84694539678223));
#4273=CARTESIAN_POINT('Ctrl Pts',(16.8984718222692,1.49999999999997,1.8691771923285));
#4274=CARTESIAN_POINT('Ctrl Pts',(16.9141139993378,1.49999999999998,1.89116874693433));
#4275=CARTESIAN_POINT('Ctrl Pts',(16.9345229122745,1.49999999999998,1.91986192188849));
#4276=CARTESIAN_POINT('Ctrl Pts',(16.9538674058155,1.49999999999999,1.9485294650334));
#4277=CARTESIAN_POINT('Ctrl Pts',(16.9723861669818,1.49999999999999,1.97724358210273));
#4278=CARTESIAN_POINT('Ctrl Pts',(16.9925517880249,1.49999999999999,2.00851122458723));
#4279=CARTESIAN_POINT('Ctrl Pts',(17.0117380772993,1.5,2.03983422915842));
#4280=CARTESIAN_POINT('Ctrl Pts',(17.0302016163928,1.5,2.07134003671764));
#4281=CARTESIAN_POINT('Ctrl Pts',(17.0507711646618,1.50000000000001,2.10643949549775));
#4282=CARTESIAN_POINT('Ctrl Pts',(17.0704434160113,1.50000000000001,2.14176601350759));
#4283=CARTESIAN_POINT('Ctrl Pts',(17.0895152061429,1.50000000000001,2.17753420398472));
#4284=CARTESIAN_POINT('Ctrl Pts',(17.1041102362821,1.50000000000001,2.2049064545411));
#4285=CARTESIAN_POINT('Ctrl Pts',(17.1183522320751,1.50000000000002,2.23253828069445));
#4286=CARTESIAN_POINT('Ctrl Pts',(17.1323574194186,1.50000000000002,2.26053700349877));
#4287=CARTESIAN_POINT('Ctrl Pts',(17.1905958043563,1.50000000000002,2.3769653208395));
#4288=CARTESIAN_POINT('Ctrl Pts',(17.2430687017406,1.50000000000001,2.49654517074463));
#4289=CARTESIAN_POINT('Ctrl Pts',(17.2937552864049,1.49999999999999,2.61706719569844));
#4290=CARTESIAN_POINT('Ctrl Pts',(17.2989790764655,1.49999999999999,2.62948826845757));
#4291=CARTESIAN_POINT('Ctrl Pts',(17.3041839329455,1.49999999999998,2.64191931324455));
#4292=CARTESIAN_POINT('Ctrl Pts',(17.3093742528659,1.49999999999998,2.65435787846686));
#4293=CARTESIAN_POINT('Ctrl Pts',(17.4414703649819,1.49999999999992,2.97092528304739));
#4294=CARTESIAN_POINT('Ctrl Pts',(17.5736371531937,1.49999999999998,3.28766206239461));
#4295=CARTESIAN_POINT('Ctrl Pts',(17.7057705722715,1.50000000000001,3.6043188728468));
#4296=CARTESIAN_POINT('Origin',(1.14001967775083,0.,4.86953436266123));
#4297=CARTESIAN_POINT('',(12.2112288551483,0.,2.96506760632555));
#4298=CARTESIAN_POINT('',(12.2112288551483,0.,2.96506760632555));
#4299=CARTESIAN_POINT('',(15.5758189333363,0.,2.23621039387092));
#4300=CARTESIAN_POINT('Origin',(12.2112288551483,0.,2.96506760632555));
#4301=CARTESIAN_POINT('',(12.2112288551483,1.13559712679391,2.96506760632555));
#4302=CARTESIAN_POINT('',(12.2112288551483,0.,2.96506760632555));
#4303=CARTESIAN_POINT('',(12.2112288551483,1.13559712679391,2.96506760632555));
#4304=CARTESIAN_POINT('Origin',(15.5758189333363,0.,2.23621039387092));
#4305=CARTESIAN_POINT('Ctrl Pts',(15.5758189333363,0.500001553330218,2.23621039387092));
#4306=CARTESIAN_POINT('Ctrl Pts',(15.5730336227227,0.500001882640314,2.23681376417234));
#4307=CARTESIAN_POINT('Ctrl Pts',(15.5702580407276,0.500018346317171,2.23741502700341));
#4308=CARTESIAN_POINT('Ctrl Pts',(15.5643001119515,0.50008718504273,2.23870566843635));
#4309=CARTESIAN_POINT('Ctrl Pts',(15.5611274155881,0.500144191417668,2.23939295650823));
#4310=CARTESIAN_POINT('Ctrl Pts',(15.5510117219381,0.500388368687124,2.24158427732426));
#4311=CARTESIAN_POINT('Ctrl Pts',(15.5440683103694,0.500649781031692,2.24308839981268));
#4312=CARTESIAN_POINT('Ctrl Pts',(15.5152010219118,0.502094399985514,2.24934180094249));
#4313=CARTESIAN_POINT('Ctrl Pts',(15.4932093723954,0.504055639212508,2.25410576088748));
#4314=CARTESIAN_POINT('Ctrl Pts',(15.2021332613909,0.538654377367701,2.31716037317271));
#4315=CARTESIAN_POINT('Ctrl Pts',(14.857471604382,0.679244250275084,2.39182300033673));
#4316=CARTESIAN_POINT('Ctrl Pts',(13.758009643497,1.01645800356828,2.62999489093509));
#4317=CARTESIAN_POINT('Ctrl Pts',(13.1844003185397,1.10083856412948,2.75425350310206));
#4318=CARTESIAN_POINT('Ctrl Pts',(12.5183408466543,1.1300613879725,2.89853920766812));
#4319=CARTESIAN_POINT('Ctrl Pts',(12.4381215277557,1.13247032707045,2.91591678645149));
#4320=CARTESIAN_POINT('Ctrl Pts',(12.3317848486809,1.13439812345724,2.93895206079133));
#4321=CARTESIAN_POINT('Ctrl Pts',(12.3054859847343,1.13477708481274,2.94464907475779));
#4322=CARTESIAN_POINT('Ctrl Pts',(12.2563519030578,1.13530868818302,2.95529278735724));
#4323=CARTESIAN_POINT('Ctrl Pts',(12.2337962495623,1.13548464416554,2.96017892514812));
#4324=CARTESIAN_POINT('Ctrl Pts',(12.2112288551483,1.13559712679392,2.96506760632553));
#4325=CARTESIAN_POINT('Ctrl Pts',(-34.0397312276251,1.50001651647932,-1.36909522182877));
#4326=CARTESIAN_POINT('Ctrl Pts',(-33.1924498698387,1.50001651647932,-0.612825791490121));
#4327=CARTESIAN_POINT('Ctrl Pts',(-32.3451685120505,1.50001651647932,0.143443638845921));
#4328=CARTESIAN_POINT('Ctrl Pts',(-31.2860668148188,1.50001651647932,1.08878042677087));
#4329=CARTESIAN_POINT('Ctrl Pts',(-31.0742464753715,1.50001651647932,1.27784778435461));
#4330=CARTESIAN_POINT('Ctrl Pts',(-30.756515966202,1.50001651647932,1.56144882073196));
#4331=CARTESIAN_POINT('Ctrl Pts',(-30.6506057964787,1.50001651647932,1.65598249952408));
#4332=CARTESIAN_POINT('Ctrl Pts',(-30.4917405418936,1.50001651647932,1.79778301771254));
#4333=CARTESIAN_POINT('Ctrl Pts',(-30.4387854570318,1.50001651647932,1.84504985710868));
#4334=CARTESIAN_POINT('Ctrl Pts',(-30.3725916009548,1.50001651647932,1.90413340635381));
#4335=CARTESIAN_POINT('Ctrl Pts',(-30.3593528297393,1.50001651647932,1.91595011620282));
#4336=CARTESIAN_POINT('Ctrl Pts',(-30.3328752873086,1.50001651647932,1.9395835359009));
#4337=CARTESIAN_POINT('Ctrl Pts',(-30.3196192754619,1.50001651647932,1.95137367689095));
#4338=CARTESIAN_POINT('Ctrl Pts',(-30.279760622108,1.50001651647932,1.98660505148068));
#4339=CARTESIAN_POINT('Ctrl Pts',(-30.2530838382129,1.50001651647932,2.00993238371371));
#4340=CARTESIAN_POINT('Ctrl Pts',(-29.7978109883261,1.50001651647932,2.40378259345705));
#4341=CARTESIAN_POINT('Ctrl Pts',(-29.3426281831049,1.50001651647932,2.73347543301461));
#4342=CARTESIAN_POINT('Ctrl Pts',(-28.3829118941348,1.50001651647932,3.31707202741814));
#4343=CARTESIAN_POINT('Ctrl Pts',(-27.8783875922888,1.50001651647932,3.57098988537781));
#4344=CARTESIAN_POINT('Ctrl Pts',(-27.0888633012187,1.50001651647932,3.90159045490631));
#4345=CARTESIAN_POINT('Ctrl Pts',(-26.8200407752322,1.50001651647932,4.00340708499724));
#4346=CARTESIAN_POINT('Ctrl Pts',(-26.2812668399142,1.50001651647932,4.1889095609928));
#4347=CARTESIAN_POINT('Ctrl Pts',(-26.0101801979463,1.50001651647932,4.27310549979575));
#4348=CARTESIAN_POINT('Ctrl Pts',(-24.6474983424516,1.50001651647932,4.65759925751976));
#4349=CARTESIAN_POINT('Ctrl Pts',(-23.5345222531661,1.50001651647932,4.85027683035403));
#4350=CARTESIAN_POINT('Ctrl Pts',(-21.8492529263652,1.50001651647932,5.05973886640617));
#4351=CARTESIAN_POINT('Ctrl Pts',(-21.2847354172308,1.50001651647932,5.11600347268612));
#4352=CARTESIAN_POINT('Ctrl Pts',(-20.1530422384387,1.50001651647932,5.21376207945505));
#4353=CARTESIAN_POINT('Ctrl Pts',(-19.5870931764672,1.50001651647932,5.25457415792074));
#4354=CARTESIAN_POINT('Ctrl Pts',(-17.8889409412059,1.50001651647932,5.35299518486675));
#4355=CARTESIAN_POINT('Ctrl Pts',(-16.7564329002056,1.50001651647932,5.38660322444038));
#4356=CARTESIAN_POINT('Ctrl Pts',(-14.4906119904705,1.50001651647932,5.39045877557458));
#4357=CARTESIAN_POINT('Ctrl Pts',(-13.3572991273454,1.50001651647932,5.36070672866599));
#4358=CARTESIAN_POINT('Ctrl Pts',(-11.6567280104122,1.50001651647932,5.26869988662586));
#4359=CARTESIAN_POINT('Ctrl Pts',(-11.08998101943,1.50001651647932,5.22990018811796));
#4360=CARTESIAN_POINT('Ctrl Pts',(-9.9585090978714,1.50001651647932,5.13906450906196));
#4361=CARTESIAN_POINT('Ctrl Pts',(-9.39348094946301,1.50001651647932,5.08709034211947));
#4362=CARTESIAN_POINT('Ctrl Pts',(-6.57095080537902,1.50001651647932,4.80303784019359));
#4363=CARTESIAN_POINT('Ctrl Pts',(-4.32119839454725,1.50001651647932,4.49917594155329));
#4364=CARTESIAN_POINT('Ctrl Pts',(-0.941769866396083,1.50001651647932,4.08783925511307));
#4365=CARTESIAN_POINT('Ctrl Pts',(0.185432109304758,1.50001651647932,3.95808364226252));
#4366=CARTESIAN_POINT('Ctrl Pts',(2.44353563975074,1.50001651647932,3.73637424342037));
#4367=CARTESIAN_POINT('Ctrl Pts',(3.5742710607959,1.50001651647932,3.64270201570121));
#4368=CARTESIAN_POINT('Ctrl Pts',(5.83512987615239,1.50001651647932,3.44911395232651));
#4369=CARTESIAN_POINT('Ctrl Pts',(6.96588483332604,1.50001651647932,3.34948547984982));
#4370=CARTESIAN_POINT('Ctrl Pts',(9.21983034667651,1.50001651647932,3.09959443172648));
#4371=CARTESIAN_POINT('Ctrl Pts',(10.3405486815635,1.50001651647932,2.95006508649919));
#4372=CARTESIAN_POINT('Ctrl Pts',(11.5857377971987,1.50001651647932,2.72045164141356));
#4373=CARTESIAN_POINT('Ctrl Pts',(11.7239082995516,1.50001651647932,2.69421641700119));
#4374=CARTESIAN_POINT('Ctrl Pts',(11.9994569735669,1.50001651647932,2.63863200974361));
#4375=CARTESIAN_POINT('Ctrl Pts',(12.1368170203099,1.50001651647932,2.60921153318681));
#4376=CARTESIAN_POINT('Ctrl Pts',(12.5468187105572,1.50001651647932,2.51278085720776));
#4377=CARTESIAN_POINT('Ctrl Pts',(12.8173110539038,1.50001651647932,2.43732295077689));
#4378=CARTESIAN_POINT('Ctrl Pts',(13.3490272719293,1.50001651647932,2.24997621492956));
#4379=CARTESIAN_POINT('Ctrl Pts',(13.6102291757378,1.50001651647932,2.13800097705185));
#4380=CARTESIAN_POINT('Ctrl Pts',(13.9302791991952,1.50001651647932,1.97266934719546));
#4381=CARTESIAN_POINT('Ctrl Pts',(13.9939729118908,1.50001651647932,1.93835975838601));
#4382=CARTESIAN_POINT('Ctrl Pts',(14.0890439919513,1.50001651647932,1.88504992700688));
#4383=CARTESIAN_POINT('Ctrl Pts',(14.1206561581996,1.50001651647932,1.86697262234482));
#4384=CARTESIAN_POINT('Ctrl Pts',(14.1837255100384,1.50001651647932,1.8302088204661));
#4385=CARTESIAN_POINT('Ctrl Pts',(14.2151762379575,1.50001651647932,1.81149697580309));
#4386=CARTESIAN_POINT('Ctrl Pts',(14.3093533352867,1.50001651647932,1.75467275956207));
#4387=CARTESIAN_POINT('Ctrl Pts',(14.3719491491779,1.50001651647932,1.71604690764134));
#4388=CARTESIAN_POINT('Ctrl Pts',(14.4974115851479,1.50001651647932,1.6398591106154));
#4389=CARTESIAN_POINT('Ctrl Pts',(14.5602712714872,1.50001651647932,1.6022698894133));
#4390=CARTESIAN_POINT('Ctrl Pts',(14.7499431421768,1.50001651647932,1.49379697508882));
#4391=CARTESIAN_POINT('Ctrl Pts',(14.8776419496855,1.50001651647932,1.42729843352251));
#4392=CARTESIAN_POINT('Ctrl Pts',(15.1416347973429,1.50001651647932,1.31719971452458));
#4393=CARTESIAN_POINT('Ctrl Pts',(15.2777376799236,1.50001651647932,1.27361438637636));
#4394=CARTESIAN_POINT('Ctrl Pts',(15.5625910875211,1.50001651647932,1.22175349312147));
#4395=CARTESIAN_POINT('Ctrl Pts',(15.7059309495787,1.50001651647932,1.21455072070237));
#4396=CARTESIAN_POINT('Ctrl Pts',(15.920927592172,1.50001651647932,1.23677953415729));
#4397=CARTESIAN_POINT('Ctrl Pts',(15.9926752933312,1.50001651647932,1.24984772075882));
#4398=CARTESIAN_POINT('Ctrl Pts',(16.131127364388,1.50001651647932,1.28656585649914));
#4399=CARTESIAN_POINT('Ctrl Pts',(16.1984885496428,1.50001651647932,1.31027639396509));
#4400=CARTESIAN_POINT('Ctrl Pts',(16.3295222008884,1.50001651647932,1.36828261273081));
#4401=CARTESIAN_POINT('Ctrl Pts',(16.3936981208766,1.50001651647932,1.40293130074928));
#4402=CARTESIAN_POINT('Ctrl Pts',(16.5149976550397,1.50001651647932,1.48074902752459));
#4403=CARTESIAN_POINT('Ctrl Pts',(16.5723029825951,1.50001651647932,1.52388264495703));
#4404=CARTESIAN_POINT('Ctrl Pts',(16.7351057716355,1.50001651647932,1.66479536878992));
#4405=CARTESIAN_POINT('Ctrl Pts',(16.8313021633667,1.50001651647932,1.77471393776967));
#4406=CARTESIAN_POINT('Ctrl Pts',(16.9969527535348,1.50001651647932,2.00760440967715));
#4407=CARTESIAN_POINT('Ctrl Pts',(17.0680061729772,1.50001651647932,2.13185112918205));
#4408=CARTESIAN_POINT('Ctrl Pts',(17.1967382089781,1.50001651647932,2.38920810011174));
#4409=CARTESIAN_POINT('Ctrl Pts',(17.2539932137629,1.50001651647932,2.52159471797806));
#4410=CARTESIAN_POINT('Ctrl Pts',(17.309389495544,1.50001651647932,2.65435151805373));
#4411=CARTESIAN_POINT('Ctrl Pts',(17.4439154500122,1.50001651647932,2.97674202276166));
#4412=CARTESIAN_POINT('Ctrl Pts',(17.5784414044805,1.50001651647932,3.29913252746959));
#4413=CARTESIAN_POINT('Ctrl Pts',(17.7129673589487,1.50001651647932,3.62152303217752));
#4414=CARTESIAN_POINT('Ctrl Pts',(-34.7056444293428,0.499999999999992,-0.623043855628343));
#4415=CARTESIAN_POINT('Ctrl Pts',(-33.8583630715561,0.499999999999992,0.133225574709989));
#4416=CARTESIAN_POINT('Ctrl Pts',(-33.0110817137697,0.499999999999992,0.889495005047924));
#4417=CARTESIAN_POINT('Ctrl Pts',(-31.9519800165362,0.499999999999992,1.83483179297088));
#4418=CARTESIAN_POINT('Ctrl Pts',(-31.7401596770896,0.499999999999992,2.02389915055542));
#4419=CARTESIAN_POINT('Ctrl Pts',(-31.4224291679196,0.499999999999992,2.30750018693225));
#4420=CARTESIAN_POINT('Ctrl Pts',(-31.3165189981963,0.499999999999992,2.40203386572442));
#4421=CARTESIAN_POINT('Ctrl Pts',(-31.1576537436113,0.499999999999992,2.54383438391295));
#4422=CARTESIAN_POINT('Ctrl Pts',(-31.1046986587496,0.499999999999992,2.59110122330912));
#4423=CARTESIAN_POINT('Ctrl Pts',(-31.0385048026725,0.499999999999992,2.6501847725542));
#4424=CARTESIAN_POINT('Ctrl Pts',(-31.0252660314571,0.499999999999992,2.66200148240322));
#4425=CARTESIAN_POINT('Ctrl Pts',(-30.9987884890263,0.499999999999992,2.68563490210131));
#4426=CARTESIAN_POINT('Ctrl Pts',(-30.9832388632707,0.499999999999992,2.69946808101334));
#4427=CARTESIAN_POINT('Ctrl Pts',(-30.9393834899522,0.499999999999992,2.73823218750993));
#4428=CARTESIAN_POINT('Ctrl Pts',(-30.9100301799479,0.499999999999992,2.7639000016916));
#4429=CARTESIAN_POINT('Ctrl Pts',(-30.4090631337961,0.499999999999992,3.19727962452407));
#4430=CARTESIAN_POINT('Ctrl Pts',(-29.9079156984876,0.499999999999992,3.56012215843322));
#4431=CARTESIAN_POINT('Ctrl Pts',(-28.8567836899866,0.499999999999992,4.19930799510662));
#4432=CARTESIAN_POINT('Ctrl Pts',(-28.3069163147731,0.499999999999992,4.475698392225));
#4433=CARTESIAN_POINT('Ctrl Pts',(-27.4539677767877,0.499999999999992,4.8328568415799));
#4434=CARTESIAN_POINT('Ctrl Pts',(-27.164747699717,0.499999999999993,4.94235355832733));
#4435=CARTESIAN_POINT('Ctrl Pts',(-26.5876684807393,0.499999999999993,5.14104472765234));
#4436=CARTESIAN_POINT('Ctrl Pts',(-26.2985764248276,0.499999999999992,5.2307936706632));
#4437=CARTESIAN_POINT('Ctrl Pts',(-24.851719466111,0.499999999999992,5.63903823819463));
#4438=CARTESIAN_POINT('Ctrl Pts',(-23.6903478434334,0.499999999999992,5.83862031478634));
#4439=CARTESIAN_POINT('Ctrl Pts',(-21.9563545557512,0.499999999999992,6.05413824694173));
#4440=CARTESIAN_POINT('Ctrl Pts',(-21.3802100145193,0.499999999999992,6.11149674921549));
#4441=CARTESIAN_POINT('Ctrl Pts',(-20.2296946994093,0.499999999999992,6.21088126116752));
#4442=CARTESIAN_POINT('Ctrl Pts',(-19.6543438808625,0.499999999999992,6.25237114523089));
#4443=CARTESIAN_POINT('Ctrl Pts',(-17.9280242560943,0.499999999999992,6.35242468975165));
#4444=CARTESIAN_POINT('Ctrl Pts',(-16.7767888220963,0.499999999999992,6.38658655078378));
#4445=CARTESIAN_POINT('Ctrl Pts',(-14.4736593465745,0.499999999999992,6.39050558666034));
#4446=CARTESIAN_POINT('Ctrl Pts',(-13.3217653084983,0.499999999999992,6.36026329011945));
#4447=CARTESIAN_POINT('Ctrl Pts',(-11.593456856115,0.499999999999992,6.26675576127116));
#4448=CARTESIAN_POINT('Ctrl Pts',(-11.0176742635534,0.499999999999931,6.22732924297478));
#4449=CARTESIAN_POINT('Ctrl Pts',(-9.87076616810186,0.500000000000054,6.13525433228844));
#4450=CARTESIAN_POINT('Ctrl Pts',(-9.29903474634851,0.499999999999992,6.08265330862635));
#4451=CARTESIAN_POINT('Ctrl Pts',(-6.44806855419954,0.499999999999992,5.79573907165103));
#4452=CARTESIAN_POINT('Ctrl Pts',(-4.19197936980058,0.499999999999992,5.49084470148195));
#4453=CARTESIAN_POINT('Ctrl Pts',(-0.825137262501205,0.499999999999992,
5.08104000571533));
#4454=CARTESIAN_POINT('Ctrl Pts',(0.293273733998886,0.499999999999993,4.95232040469897));
#4455=CARTESIAN_POINT('Ctrl Pts',(2.5311253192372,0.499999999999993,4.73259942190914));
#4456=CARTESIAN_POINT('Ctrl Pts',(3.65773355433088,0.499999999999869,4.6392312433788));
#4457=CARTESIAN_POINT('Ctrl Pts',(5.92229763284814,0.500000000000115,4.44532591472657));
#4458=CARTESIAN_POINT('Ctrl Pts',(7.0608573913797,0.500000000000238,4.34509976949567));
#4459=CARTESIAN_POINT('Ctrl Pts',(9.34524764280534,0.499999999999746,4.09183336732117));
#4460=CARTESIAN_POINT('Ctrl Pts',(10.4885105555597,0.500000000000114,3.93965728369929));
#4461=CARTESIAN_POINT('Ctrl Pts',(11.7712568966956,0.499999999999977,3.70311827029293));
#4462=CARTESIAN_POINT('Ctrl Pts',(11.9138517815751,0.499999999999993,3.67606050201731));
#4463=CARTESIAN_POINT('Ctrl Pts',(12.2049990926623,0.499999999999993,3.61732950098476));
#4464=CARTESIAN_POINT('Ctrl Pts',(12.3527978405267,0.500000000000007,3.58571697834473));
#4465=CARTESIAN_POINT('Ctrl Pts',(12.8017143158579,0.499999999999962,3.48013371530843));
#4466=CARTESIAN_POINT('Ctrl Pts',(13.1087015369894,0.499999999999961,3.39492840425144));
#4467=CARTESIAN_POINT('Ctrl Pts',(13.7222853032534,0.500000000000023,3.17873617812773));
#4468=CARTESIAN_POINT('Ctrl Pts',(14.0281358746551,0.499999999999961,3.04768383691634));
#4469=CARTESIAN_POINT('Ctrl Pts',(14.3995116112702,0.5,2.8558383396111));
#4470=CARTESIAN_POINT('Ctrl Pts',(14.473269524189,0.5,2.81610352931213));
#4471=CARTESIAN_POINT('Ctrl Pts',(14.5830463690884,0.499999999999988,2.75454763752365));
#4472=CARTESIAN_POINT('Ctrl Pts',(14.6194957575626,0.499999999999988,2.73370357088325));
#4473=CARTESIAN_POINT('Ctrl Pts',(14.6920997332583,0.499999999999996,2.69138193423077));
#4474=CARTESIAN_POINT('Ctrl Pts',(14.7287241088115,0.499999999999992,2.66958471801292));
#4475=CARTESIAN_POINT('Ctrl Pts',(14.8321427204664,0.499999999999992,2.60718437024267));
#4476=CARTESIAN_POINT('Ctrl Pts',(14.8947429371819,0.499999999999992,2.56853667987705));
#4477=CARTESIAN_POINT('Ctrl Pts',(15.0127324953208,0.499999999999992,2.49688681601923));
#4478=CARTESIAN_POINT('Ctrl Pts',(15.0679261119592,0.499999999999992,2.46394621747195));
#4479=CARTESIAN_POINT('Ctrl Pts',(15.2239960512198,0.499999999999992,2.37469015503045));
#4480=CARTESIAN_POINT('Ctrl Pts',(15.3151397369363,0.500000000000023,2.32833861119067));
#4481=CARTESIAN_POINT('Ctrl Pts',(15.4739865129508,0.499999999999961,2.26209124628497));
#4482=CARTESIAN_POINT('Ctrl Pts',(15.5412102426098,0.499999999999976,2.24210104315146));
#4483=CARTESIAN_POINT('Ctrl Pts',(15.6573592971275,0.500000000000008,2.22095473893486));
#4484=CARTESIAN_POINT('Ctrl Pts',(15.7044313152833,0.499999999999992,2.21974296559136));
#4485=CARTESIAN_POINT('Ctrl Pts',(15.767410117571,0.499999999999992,2.22625443129171));
#4486=CARTESIAN_POINT('Ctrl Pts',(15.787122043338,0.499999999999985,2.2299203684438));
#4487=CARTESIAN_POINT('Ctrl Pts',(15.8239859664479,0.5,2.23969685326193));
#4488=CARTESIAN_POINT('Ctrl Pts',(15.84126845336,0.5,2.24576246549322));
#4489=CARTESIAN_POINT('Ctrl Pts',(15.8771446395265,0.499999999999984,2.26164420179718));
#4490=CARTESIAN_POINT('Ctrl Pts',(15.8955951643463,0.5,2.27149430071215));
#4491=CARTESIAN_POINT('Ctrl Pts',(15.9331444677752,0.499999999999985,2.2955834436242));
#4492=CARTESIAN_POINT('Ctrl Pts',(15.952275277354,0.499999999999992,2.3098037266637));
#4493=CARTESIAN_POINT('Ctrl Pts',(16.0117937275615,0.499999999999992,2.36131947594947));
#4494=CARTESIAN_POINT('Ctrl Pts',(16.0546868722937,0.499999999999992,2.40816900698943));
#4495=CARTESIAN_POINT('Ctrl Pts',(16.1437612346005,0.499999999999992,2.53339991517352));
#4496=CARTESIAN_POINT('Ctrl Pts',(16.190212071248,0.499999999999992,2.6123539981433));
#4497=CARTESIAN_POINT('Ctrl Pts',(16.2857972214586,0.499999999999992,2.80344480969631));
#4498=CARTESIAN_POINT('Ctrl Pts',(16.3343667769681,0.499999999999992,2.91452246837103));
#4499=CARTESIAN_POINT('Ctrl Pts',(16.386497303637,0.499999999999992,3.03945284932728));
#4500=CARTESIAN_POINT('Ctrl Pts',(16.5130926026644,0.499999999999992,3.34283744843543));
#4501=CARTESIAN_POINT('Ctrl Pts',(16.6396879016917,0.499999999999992,3.64622204754358));
#4502=CARTESIAN_POINT('Ctrl Pts',(16.766283200719,0.499999999999992,3.94960664665173));
#4503=CARTESIAN_POINT('Ctrl Pts',(-34.7123034513764,0.489999999999992,-0.615583465185726));
#4504=CARTESIAN_POINT('Ctrl Pts',(-33.8650220935896,0.489999999999992,0.140685965152536));
#4505=CARTESIAN_POINT('Ctrl Pts',(-33.0177407358033,0.489999999999992,0.896955395490548));
#4506=CARTESIAN_POINT('Ctrl Pts',(-31.9586390385697,0.489999999999992,1.84229218341346));
#4507=CARTESIAN_POINT('Ctrl Pts',(-31.7468186991232,0.489999999999992,2.03135954099803));
#4508=CARTESIAN_POINT('Ctrl Pts',(-31.4290881899532,0.489999999999992,2.31496057737484));
#4509=CARTESIAN_POINT('Ctrl Pts',(-31.3231780202299,0.489999999999992,2.40949425616707));
#4510=CARTESIAN_POINT('Ctrl Pts',(-31.1643127656449,0.489999999999992,2.55129477435557));
#4511=CARTESIAN_POINT('Ctrl Pts',(-31.1113576807832,0.489999999999992,2.59856161375176));
#4512=CARTESIAN_POINT('Ctrl Pts',(-31.0451638247061,0.489999999999992,2.65764516299682));
#4513=CARTESIAN_POINT('Ctrl Pts',(-31.0319250534907,0.489999999999992,2.66946187284586));
#4514=CARTESIAN_POINT('Ctrl Pts',(-31.0054475110599,0.489999999999992,2.69309529254392));
#4515=CARTESIAN_POINT('Ctrl Pts',(-30.9898749495441,0.489999999999992,2.70694890149773));
#4516=CARTESIAN_POINT('Ctrl Pts',(-30.945979609686,0.489999999999992,2.74574833473001));
#4517=CARTESIAN_POINT('Ctrl Pts',(-30.9165995348626,0.489999999999991,2.7714395533445));
#4518=CARTESIAN_POINT('Ctrl Pts',(-30.4151755542951,0.489999999999991,3.20521446377914));
#4519=CARTESIAN_POINT('Ctrl Pts',(-29.9135684802773,0.489999999999992,3.5683884891567));
#4520=CARTESIAN_POINT('Ctrl Pts',(-28.8615223296795,0.489999999999992,4.2081302090716));
#4521=CARTESIAN_POINT('Ctrl Pts',(-28.3112015312213,0.489999999999992,4.48474532786999));
#4522=CARTESIAN_POINT('Ctrl Pts',(-27.457618761242,0.489999999999992,4.84216935163674));
#4523=CARTESIAN_POINT('Ctrl Pts',(-27.1681947120293,0.489999999999992,4.9517428679823));
#4524=CARTESIAN_POINT('Ctrl Pts',(-26.5907324465417,0.489999999999992,5.15056592206242));
#4525=CARTESIAN_POINT('Ctrl Pts',(-26.3014603394644,0.489999999999992,5.24037039419811));
#4526=CARTESIAN_POINT('Ctrl Pts',(-24.8537616436179,0.489999999999992,5.64885246590485));
#4527=CARTESIAN_POINT('Ctrl Pts',(-23.6919060735996,0.489999999999992,5.8485035863938));
#4528=CARTESIAN_POINT('Ctrl Pts',(-21.957425554356,0.489999999999992,6.06408207651008));
#4529=CARTESIAN_POINT('Ctrl Pts',(-21.3811647447234,0.489999999999992,6.12145151756312));
#4530=CARTESIAN_POINT('Ctrl Pts',(-20.230461211359,0.489999999999992,6.22085228829844));
#4531=CARTESIAN_POINT('Ctrl Pts',(-19.6550163767992,0.489999999999992,6.26234895030581));
#4532=CARTESIAN_POINT('Ctrl Pts',(-17.9284150827881,0.489999999999992,6.36241881973267));
#4533=CARTESIAN_POINT('Ctrl Pts',(-16.7769923779532,0.489999999999992,6.3965862188879));
#4534=CARTESIAN_POINT('Ctrl Pts',(-14.4734898229355,0.489999999999992,6.40050588960137));
#4535=CARTESIAN_POINT('Ctrl Pts',(-13.3214099761787,0.489999999999992,6.37025869064512));
#4536=CARTESIAN_POINT('Ctrl Pts',(-11.592824155022,0.489999999999992,6.27673615517661));
#4537=CARTESIAN_POINT('Ctrl Pts',(-11.016951207937,0.48999999999993,6.2373033687859));
#4538=CARTESIAN_POINT('Ctrl Pts',(-9.86988875329596,0.490000000000055,6.14521606598797));
#4539=CARTESIAN_POINT('Ctrl Pts',(-9.29809029991629,0.489999999999992,6.0926087738622));
#4540=CARTESIAN_POINT('Ctrl Pts',(-6.44683975198322,0.489999999999992,5.80566592000903));
#4541=CARTESIAN_POINT('Ctrl Pts',(-4.19068720089519,0.489999999999992,5.50076122529517));
#4542=CARTESIAN_POINT('Ctrl Pts',(-0.823970955725548,0.489999999999992,
5.09097184918228));
#4543=CARTESIAN_POINT('Ctrl Pts',(0.294352132434478,0.489999999999992,4.96226260811314));
#4544=CARTESIAN_POINT('Ctrl Pts',(2.53200120156563,0.489999999999992,4.7425615091555));
#4545=CARTESIAN_POINT('Ctrl Pts',(3.65856816548137,0.489999999999868,4.64919637106674));
#4546=CARTESIAN_POINT('Ctrl Pts',(5.92316929601833,0.490000000000116,4.45528786981418));
#4547=CARTESIAN_POINT('Ctrl Pts',(7.06180710127438,0.49000000000024,4.35505574795442));
#4548=CARTESIAN_POINT('Ctrl Pts',(9.34650179505245,0.489999999999744,4.1017555927969));
#4549=CARTESIAN_POINT('Ctrl Pts',(10.489990149862,0.490000000000115,3.9495530422282));
#4550=CARTESIAN_POINT('Ctrl Pts',(11.7731120570498,0.489999999999977,3.7129447742825));
#4551=CARTESIAN_POINT('Ctrl Pts',(11.9157511850239,0.489999999999992,3.68587878070408));
#4552=CARTESIAN_POINT('Ctrl Pts',(12.2070544799055,0.489999999999992,3.62711631425347));
#4553=CARTESIAN_POINT('Ctrl Pts',(12.3549576130571,0.490000000000008,3.59548187151465));
#4554=CARTESIAN_POINT('Ctrl Pts',(12.8042632298119,0.489999999999962,3.48980708411944));
#4555=CARTESIAN_POINT('Ctrl Pts',(13.1116153936936,0.489999999999961,3.40450430062607));
#4556=CARTESIAN_POINT('Ctrl Pts',(13.7260178219185,0.490000000000023,3.1880236243638));
#4557=CARTESIAN_POINT('Ctrl Pts',(14.0323148726219,0.48999999999996,3.05678051526989));
#4558=CARTESIAN_POINT('Ctrl Pts',(14.4042038578915,0.49,2.86466988366926));
#4559=CARTESIAN_POINT('Ctrl Pts',(14.4780624111504,0.49,2.82488082205141));
#4560=CARTESIAN_POINT('Ctrl Pts',(14.5879863112693,0.489999999999988,2.7632424710208));
#4561=CARTESIAN_POINT('Ctrl Pts',(14.6244840711669,0.489999999999988,2.74237073721757));
#4562=CARTESIAN_POINT('Ctrl Pts',(14.6971833915264,0.489999999999997,2.69999352313528));
#4563=CARTESIAN_POINT('Ctrl Pts',(14.7338595027015,0.489999999999992,2.67816545371149));
#4564=CARTESIAN_POINT('Ctrl Pts',(14.8373705279732,0.489999999999992,2.61570934554691));
#4565=CARTESIAN_POINT('Ctrl Pts',(14.8999707887162,0.489999999999992,2.57706143680043));
#4566=CARTESIAN_POINT('Ctrl Pts',(15.0178856193111,0.489999999999992,2.50545695152482));
#4567=CARTESIAN_POINT('Ctrl Pts',(15.0730025765186,0.489999999999992,2.47256283843628));
#4568=CARTESIAN_POINT('Ctrl Pts',(15.2287365020147,0.489999999999992,2.38349894133971));
#4569=CARTESIAN_POINT('Ctrl Pts',(15.3195146425508,0.490000000000023,2.33734886414972));
#4570=CARTESIAN_POINT('Ctrl Pts',(15.477309975215,0.489999999999961,2.27154000554233));
#4571=CARTESIAN_POINT('Ctrl Pts',(15.543844924721,0.489999999999977,2.25178574976194));
#4572=CARTESIAN_POINT('Ctrl Pts',(15.6583069635714,0.490000000000008,2.23094658636282));
#4573=CARTESIAN_POINT('Ctrl Pts',(15.704416319188,0.489999999999992,2.22979472202062));
#4574=CARTESIAN_POINT('Ctrl Pts',(15.7658749681803,0.489999999999992,2.23614901683935));
#4575=CARTESIAN_POINT('Ctrl Pts',(15.7850665447876,0.489999999999984,2.23972093304985));
#4576=CARTESIAN_POINT('Ctrl Pts',(15.8209146031966,0.49,2.24922800580848));
#4577=CARTESIAN_POINT('Ctrl Pts',(15.8376963113963,0.49,2.25511717170168));
#4578=CARTESIAN_POINT('Ctrl Pts',(15.8726209386285,0.489999999999984,2.2705776701384));
#4579=CARTESIAN_POINT('Ctrl Pts',(15.8906142170488,0.49,2.28017978725815));
#4580=CARTESIAN_POINT('Ctrl Pts',(15.9273260320027,0.489999999999984,2.30373165320545));
#4581=CARTESIAN_POINT('Ctrl Pts',(15.9460751027066,0.489999999999992,2.31766280767642));
#4582=CARTESIAN_POINT('Ctrl Pts',(16.0045607265845,0.489999999999992,2.36828460198171));
#4583=CARTESIAN_POINT('Ctrl Pts',(16.0469208476503,0.489999999999992,2.41450345305888));
#4584=CARTESIAN_POINT('Ctrl Pts',(16.135229460326,0.489999999999992,2.53865778338701));
#4585=CARTESIAN_POINT('Ctrl Pts',(16.181434275209,0.489999999999992,2.61715894747207));
#4586=CARTESIAN_POINT('Ctrl Pts',(16.2766879620364,0.489999999999992,2.80758710837596));
#4587=CARTESIAN_POINT('Ctrl Pts',(16.3251706644875,0.489999999999992,2.91845168097819));
#4588=CARTESIAN_POINT('Ctrl Pts',(16.3772685341448,0.489999999999992,3.04330379903588));
#4589=CARTESIAN_POINT('Ctrl Pts',(16.5037845279275,0.489999999999992,3.34649834222707));
#4590=CARTESIAN_POINT('Ctrl Pts',(16.6303005217103,0.489999999999992,3.64969288541828));
#4591=CARTESIAN_POINT('Ctrl Pts',(16.756816515493,0.489999999999992,3.95288742860948));
#12113=UNCERTAINTY_MEASURE_WITH_UNIT(LENGTH_MEASURE(0.01),#12138,
'DISTANCE_ACCURACY_VALUE',
'Maximum model space distance between geometric entities at asserted c
onnectivities');
#12123=UNCERTAINTY_MEASURE_WITH_UNIT(LENGTH_MEASURE(0.01),#12138,
'DISTANCE_ACCURACY_VALUE',
'Maximum model space distance between geometric entities at asserted c
onnectivities');
#12127=(
GEOMETRIC_REPRESENTATION_CONTEXT(3)
GLOBAL_UNCERTAINTY_ASSIGNED_CONTEXT((#12113))
GLOBAL_UNIT_ASSIGNED_CONTEXT((#12138,#12140,#12141))
REPRESENTATION_CONTEXT('','3D')
);
#12137=(
GEOMETRIC_REPRESENTATION_CONTEXT(3)
GLOBAL_UNCERTAINTY_ASSIGNED_CONTEXT((#12123))
GLOBAL_UNIT_ASSIGNED_CONTEXT((#12138,#12140,#12141))
REPRESENTATION_CONTEXT('','3D')
);
#12138=(
LENGTH_UNIT()
NAMED_UNIT(*)
SI_UNIT(.MILLI.,.METRE.)
);
#12140=(
NAMED_UNIT(*)
PLANE_ANGLE_UNIT()
SI_UNIT($,.RADIAN.)
);
#12141=(
NAMED_UNIT(*)
SI_UNIT($,.STERADIAN.)
SOLID_ANGLE_UNIT()
);
#12145=SHAPE_DEFINITION_REPRESENTATION(#12158,#12186);
#12158=PRODUCT_DEFINITION_SHAPE('',$,#12200);
#12186=SHAPE_REPRESENTATION('',(#2005),#12127);
#12196=PRODUCT_DEFINITION_CONTEXT('part definition',#12237,'design');
#12200=PRODUCT_DEFINITION('knife smal','Knife small',#12213,#12196);
#12213=PRODUCT_DEFINITION_FORMATION('',$,#12242);
#12237=APPLICATION_CONTEXT(
'Core Data for Automotive Mechanical Design Process');
#12238=PRODUCT_CONTEXT('part definition',#12237,'mechanical');
#12242=PRODUCT('knife smal','Knife small',$,(#12238));
#12253=PRESENTATION_STYLE_ASSIGNMENT((#12255));
#12255=SURFACE_STYLE_USAGE(.BOTH.,#12257);
#12257=SURFACE_SIDE_STYLE('',(#12259));
#12259=SURFACE_STYLE_FILL_AREA(#12261);
#12261=FILL_AREA_STYLE('Opaque(23,69,131)',(#12263));
#12263=FILL_AREA_STYLE_COLOUR('Opaque(23,69,131)',#12265);
#12265=COLOUR_RGB('Opaque(23,69,131)',0.0901960784313725,0.270588235294118,
0.513725490196078);
ENDSEC;
END-ISO-10303-21;
